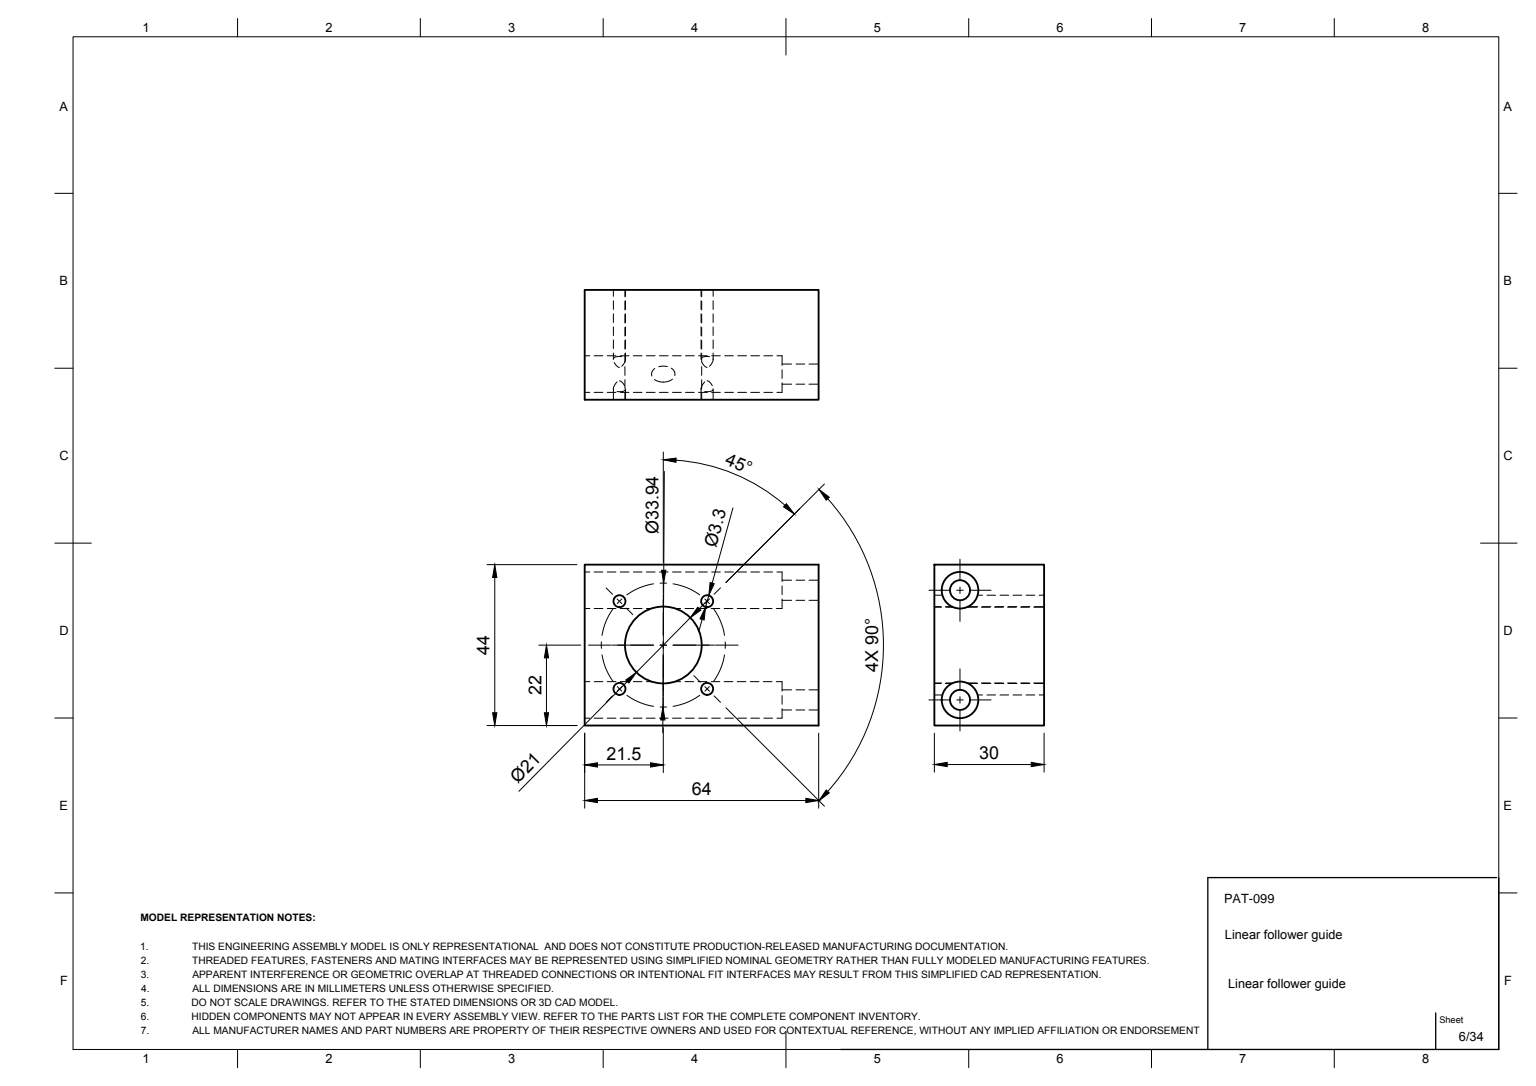
ISO-10303-21;
HEADER;
/* Generated by software containing ST-Developer
 * from STEP Tools, Inc. (www.steptools.com) 
 */

FILE_DESCRIPTION(
/* description */ ('PAT-099'),
/* implementation_level */ '2;1');

FILE_NAME(
/* name */ 'Linear follower guide.step',
/* time_stamp */ '2026-10-29T17:25:42-07:00',
/* author */ (''),
/* organization */ (''),
/* preprocessor_version */ 'ST-DEVELOPER v20.2',
/* originating_system */ 'Autodesk Translation Framework v15.17.0.0',
/* authorisation */ '');

FILE_SCHEMA (('AUTOMOTIVE_DESIGN { 1 0 10303 214 3 1 1 }'));
ENDSEC;

DATA;
#10=MECHANICAL_DESIGN_GEOMETRIC_PRESENTATION_REPRESENTATION('',(#338),#11035);
#241=B_SPLINE_CURVE_WITH_KNOTS('',3,(#7321,#7322,#7323,#7324,#7325,#7326,
#7327,#7328,#7329,#7330,#7331,#7332,#7333,#7334,#7335,#7336,#7337,#7338,
#7339,#7340,#7341,#7342,#7343,#7344,#7345,#7346,#7347,#7348,#7349,#7350),
 .UNSPECIFIED.,.F.,.F.,(4,2,2,2,2,2,2,2,2,2,2,2,2,2,4),(0.,0.0614386993115687,
0.122877398623137,0.194452004299172,0.266026609975207,0.361453659820112,
0.456880709665017,0.528368337752035,0.564112151795545,0.599855965839054,
0.635599779882563,0.671343593926072,0.742831222013091,0.838258271857996,
0.933685321702901),.UNSPECIFIED.);
#242=B_SPLINE_CURVE_WITH_KNOTS('',3,(#7351,#7352,#7353,#7354,#7355,#7356,
#7357,#7358,#7359,#7360),.UNSPECIFIED.,.F.,.F.,(4,2,2,2,4),(0.933685321702901,
1.00525992737894,1.07683453305497,1.13827323236654,1.19971193167811),
 .UNSPECIFIED.);
#243=B_SPLINE_CURVE_WITH_KNOTS('',3,(#7364,#7365,#7366,#7367,#7368,#7369,
#7370,#7371,#7372,#7373),.UNSPECIFIED.,.F.,.F.,(4,2,2,2,4),(0.,0.061438699311569,
0.122877398623138,0.194452004299173,0.266026609975207),.UNSPECIFIED.);
#244=B_SPLINE_CURVE_WITH_KNOTS('',3,(#7374,#7375,#7376,#7377,#7378,#7379,
#7380,#7381,#7382,#7383,#7384,#7385,#7386,#7387,#7388,#7389,#7390,#7391,
#7392,#7393,#7394,#7395,#7396,#7397,#7398,#7399,#7400,#7401,#7402,#7403),
 .UNSPECIFIED.,.F.,.F.,(4,2,2,2,2,2,2,2,2,2,2,2,2,2,4),(0.266026609975207,
0.361453659820112,0.456880709665017,0.528368337752036,0.564112151795545,
0.599855965839054,0.635599779882563,0.671343593926073,0.742831222013091,
0.838258271857996,0.933685321702901,1.00525992737894,1.07683453305497,1.13827323236654,
1.19971193167811),.UNSPECIFIED.);
#245=B_SPLINE_CURVE_WITH_KNOTS('',3,(#7413,#7414,#7415,#7416,#7417,#7418,
#7419,#7420,#7421,#7422,#7423,#7424,#7425,#7426,#7427,#7428,#7429,#7430,
#7431,#7432,#7433,#7434,#7435,#7436,#7437,#7438,#7439,#7440),
 .UNSPECIFIED.,.F.,.F.,(4,2,2,2,2,2,2,2,2,2,2,2,2,4),(0.,0.028138639371576,
0.0562772787431521,0.154843288866037,0.240109193198138,0.325375097530239,
0.395403587057064,0.46543207658389,0.528409281202622,0.591386485821355,
0.652825185132924,0.714263884444493,0.785838490120527,0.857413095796562),
 .UNSPECIFIED.);
#246=B_SPLINE_CURVE_WITH_KNOTS('',3,(#7441,#7442,#7443,#7444,#7445,#7446,
#7447,#7448,#7449,#7450,#7451,#7452),.UNSPECIFIED.,.F.,.F.,(4,2,2,2,2,4),
(0.857413095796562,0.952840145641466,1.04826719548637,1.11975482357339,
1.1554986376169,1.19124245166041),.UNSPECIFIED.);
#247=B_SPLINE_CURVE_WITH_KNOTS('',3,(#7456,#7457,#7458,#7459,#7460,#7461,
#7462,#7463,#7464,#7465,#7466,#7467),.UNSPECIFIED.,.F.,.F.,(4,2,2,2,2,4),
(0.,0.0357438140435093,0.0714876280870186,0.142975256174037,0.238402306018942,
0.333829355863846),.UNSPECIFIED.);
#248=B_SPLINE_CURVE_WITH_KNOTS('',3,(#7468,#7469,#7470,#7471,#7472,#7473,
#7474,#7475,#7476,#7477,#7478,#7479,#7480,#7481,#7482,#7483,#7484,#7485,
#7486,#7487,#7488,#7489,#7490,#7491,#7492,#7493,#7494,#7495),
 .UNSPECIFIED.,.F.,.F.,(4,2,2,2,2,2,2,2,2,2,2,2,2,4),(0.333829355863846,
0.40540396153988,0.476978567215915,0.538417266527484,0.599855965839053,
0.662833170457785,0.725810375076518,0.795838864603343,0.865867354130168,
0.951133258462269,1.03639916279437,1.13496517291726,1.16310381228883,1.19124245166041),
 .UNSPECIFIED.);
#249=B_SPLINE_CURVE_WITH_KNOTS('',3,(#7505,#7506,#7507,#7508,#7509,#7510,
#7511,#7512,#7513,#7514,#7515,#7516,#7517,#7518,#7519,#7520,#7521,#7522,
#7523,#7524,#7525,#7526,#7527,#7528,#7529,#7530,#7531,#7532),
 .UNSPECIFIED.,.F.,.F.,(4,2,2,2,2,2,2,2,2,2,2,2,2,4),(0.,0.0357438140435092,
0.0714876280870185,0.142975256174037,0.238402306018942,0.333829355863847,
0.405403961539882,0.476978567215916,0.538417266527485,0.599855965839054,
0.661294665150623,0.722733364462192,0.794307970138227,0.865882575814261),
 .UNSPECIFIED.);
#250=B_SPLINE_CURVE_WITH_KNOTS('',3,(#7533,#7534,#7535,#7536,#7537,#7538,
#7539,#7540,#7541,#7542,#7543,#7544),.UNSPECIFIED.,.F.,.F.,(4,2,2,2,2,4),
(0.865882575814261,0.961309625659166,1.05673667550407,1.12822430359109,
1.1639681176346,1.19971193167811),.UNSPECIFIED.);
#251=B_SPLINE_CURVE_WITH_KNOTS('',3,(#7548,#7549,#7550,#7551,#7552,#7553,
#7554,#7555,#7556,#7557,#7558,#7559),.UNSPECIFIED.,.F.,.F.,(4,2,2,2,2,4),
(0.,0.0357438140435093,0.0714876280870185,0.142975256174037,0.238402306018942,
0.333829355863847),.UNSPECIFIED.);
#252=B_SPLINE_CURVE_WITH_KNOTS('',3,(#7560,#7561,#7562,#7563,#7564,#7565,
#7566,#7567,#7568,#7569,#7570,#7571,#7572,#7573,#7574,#7575,#7576,#7577,
#7578,#7579,#7580,#7581,#7582,#7583,#7584,#7585,#7586,#7587),
 .UNSPECIFIED.,.F.,.F.,(4,2,2,2,2,2,2,2,2,2,2,2,2,4),(0.333829355863847,
0.405403961539881,0.476978567215916,0.538417266527485,0.599855965839054,
0.661294665150623,0.722733364462191,0.794307970138226,0.865882575814261,
0.961309625659166,1.05673667550407,1.12822430359109,1.1639681176346,1.19971193167811),
 .UNSPECIFIED.);
#253=B_SPLINE_CURVE_WITH_KNOTS('',3,(#7597,#7598,#7599,#7600,#7601,#7602,
#7603,#7604,#7605,#7606,#7607,#7608,#7609,#7610,#7611,#7612,#7613,#7614,
#7615,#7616,#7617,#7618,#7619,#7620,#7621,#7622,#7623,#7624,#7625,#7626),
 .UNSPECIFIED.,.F.,.F.,(4,2,2,2,2,2,2,2,2,2,2,2,2,2,4),(0.,0.0629772046187326,
0.125954409237465,0.195982898764291,0.266011388291116,0.351277292623217,
0.436543196955317,0.535109207078203,0.563247846449779,0.591386485821355,
0.627130299864864,0.662874113908373,0.734361741995392,0.829788791840296,
0.925215841685201),.UNSPECIFIED.);
#254=B_SPLINE_CURVE_WITH_KNOTS('',3,(#7627,#7628,#7629,#7630,#7631,#7632,
#7633,#7634,#7635,#7636),.UNSPECIFIED.,.F.,.F.,(4,2,2,2,4),(0.925215841685201,
0.996790447361235,1.06836505303727,1.12980375234884,1.19124245166041),
 .UNSPECIFIED.);
#255=B_SPLINE_CURVE_WITH_KNOTS('',3,(#7640,#7641,#7642,#7643,#7644,#7645,
#7646,#7647,#7648,#7649),.UNSPECIFIED.,.F.,.F.,(4,2,2,2,4),(0.,0.061438699311569,
0.122877398623138,0.194452004299172,0.266026609975207),.UNSPECIFIED.);
#256=B_SPLINE_CURVE_WITH_KNOTS('',3,(#7650,#7651,#7652,#7653,#7654,#7655,
#7656,#7657,#7658,#7659,#7660,#7661,#7662,#7663,#7664,#7665,#7666,#7667,
#7668,#7669,#7670,#7671,#7672,#7673,#7674,#7675,#7676,#7677,#7678,#7679),
 .UNSPECIFIED.,.F.,.F.,(4,2,2,2,2,2,2,2,2,2,2,2,2,2,4),(0.266026609975207,
0.361453659820111,0.456880709665016,0.528368337752034,0.564112151795544,
0.599855965839053,0.627994605210629,0.656133244582205,0.75469925470509,
0.839965159037191,0.925231063369292,0.995259552896117,1.06528804242294,
1.12826524704167,1.19124245166041),.UNSPECIFIED.);
#257=B_SPLINE_CURVE_WITH_KNOTS('',3,(#7688,#7689,#7690,#7691,#7692,#7693,
#7694,#7695,#7696,#7697,#7698,#7699,#7700,#7701,#7702,#7703,#7704,#7705,
#7706,#7707,#7708,#7709,#7710,#7711,#7712,#7713,#7714,#7715,#7716,#7717,
#7718,#7719,#7720,#7721,#7722,#7723,#7724,#7725,#7726,#7727,#7728,#7729),
 .UNSPECIFIED.,.T.,.F.,(4,2,2,2,2,2,2,2,2,2,2,2,2,2,2,2,2,2,2,2,4),(0.,
0.157447434703095,0.236171152054642,0.314894869406189,0.367076252690622,
0.419257635975055,0.471439019259488,0.523620402543921,0.602344119895468,
0.681067837247015,0.83851527195011,0.995962706653205,1.07468642400475,1.1534101413563,
1.20559152464073,1.25777290792516,1.3099542912096,1.36213567449403,1.44085939184558,
1.51958310919713,1.67703054390022),.UNSPECIFIED.);
#258=B_SPLINE_CURVE_WITH_KNOTS('',3,(#7742,#7743,#7744,#7745,#7746,#7747,
#7748,#7749,#7750,#7751,#7752,#7753,#7754,#7755,#7756,#7757,#7758,#7759,
#7760,#7761,#7762,#7763,#7764,#7765,#7766,#7767,#7768,#7769,#7770,#7771,
#7772,#7773,#7774,#7775,#7776,#7777,#7778,#7779,#7780,#7781,#7782,#7783),
 .UNSPECIFIED.,.T.,.F.,(4,2,2,2,2,2,2,2,2,2,2,2,2,2,2,2,2,2,2,2,4),(0.,
0.157447434703095,0.236171152054642,0.314894869406189,0.367076252690622,
0.419257635975055,0.471439019259488,0.523620402543921,0.602344119895468,
0.681067837247015,0.83851527195011,0.995962706653205,1.07468642400475,1.1534101413563,
1.20559152464073,1.25777290792516,1.3099542912096,1.36213567449403,1.44085939184558,
1.51958310919713,1.67703054390022),.UNSPECIFIED.);
#288=SHAPE_REPRESENTATION_RELATIONSHIP('SRR','None',#11156,#313);
#313=ADVANCED_BREP_SHAPE_REPRESENTATION('',(#371),#11006);
#338=STYLED_ITEM('',(#11400),#371);
#371=MANIFOLD_SOLID_BREP('Body1',#4706);
#413=FACE_BOUND('',#965,.T.);
#414=FACE_BOUND('',#966,.T.);
#415=FACE_BOUND('',#978,.T.);
#416=FACE_BOUND('',#979,.T.);
#417=FACE_BOUND('',#980,.T.);
#418=FACE_BOUND('',#981,.T.);
#419=FACE_BOUND('',#982,.T.);
#420=FACE_BOUND('',#984,.T.);
#421=FACE_BOUND('',#987,.T.);
#422=FACE_BOUND('',#988,.T.);
#423=FACE_BOUND('',#989,.T.);
#424=FACE_BOUND('',#990,.T.);
#425=FACE_BOUND('',#991,.T.);
#426=FACE_BOUND('',#993,.T.);
#427=FACE_BOUND('',#996,.T.);
#428=FACE_BOUND('',#997,.T.);
#429=FACE_BOUND('',#999,.T.);
#430=FACE_BOUND('',#1000,.T.);
#431=FACE_BOUND('',#1001,.T.);
#432=FACE_BOUND('',#1002,.T.);
#433=FACE_BOUND('',#1003,.T.);
#434=FACE_BOUND('',#1005,.T.);
#435=FACE_BOUND('',#1006,.T.);
#436=FACE_BOUND('',#1007,.T.);
#437=FACE_BOUND('',#1008,.T.);
#438=FACE_BOUND('',#1009,.T.);
#439=FACE_BOUND('',#1011,.T.);
#440=FACE_BOUND('',#1012,.T.);
#529=PLANE('',#5044);
#530=PLANE('',#5047);
#531=PLANE('',#5048);
#532=PLANE('',#5067);
#533=PLANE('',#5073);
#534=PLANE('',#5080);
#535=PLANE('',#5081);
#536=PLANE('',#5082);
#671=FACE_OUTER_BOUND('',#964,.T.);
#672=FACE_OUTER_BOUND('',#967,.T.);
#673=FACE_OUTER_BOUND('',#968,.T.);
#674=FACE_OUTER_BOUND('',#969,.T.);
#675=FACE_OUTER_BOUND('',#970,.T.);
#676=FACE_OUTER_BOUND('',#971,.T.);
#677=FACE_OUTER_BOUND('',#972,.T.);
#678=FACE_OUTER_BOUND('',#973,.T.);
#679=FACE_OUTER_BOUND('',#974,.T.);
#680=FACE_OUTER_BOUND('',#975,.T.);
#681=FACE_OUTER_BOUND('',#976,.T.);
#682=FACE_OUTER_BOUND('',#977,.T.);
#683=FACE_OUTER_BOUND('',#983,.T.);
#684=FACE_OUTER_BOUND('',#985,.T.);
#685=FACE_OUTER_BOUND('',#986,.T.);
#686=FACE_OUTER_BOUND('',#992,.T.);
#687=FACE_OUTER_BOUND('',#994,.T.);
#688=FACE_OUTER_BOUND('',#995,.T.);
#689=FACE_OUTER_BOUND('',#998,.T.);
#690=FACE_OUTER_BOUND('',#1004,.T.);
#691=FACE_OUTER_BOUND('',#1010,.T.);
#964=EDGE_LOOP('',(#3191,#3192,#3193,#3194));
#965=EDGE_LOOP('',(#3195));
#966=EDGE_LOOP('',(#3196));
#967=EDGE_LOOP('',(#3197,#3198,#3199,#3200));
#968=EDGE_LOOP('',(#3201,#3202,#3203,#3204));
#969=EDGE_LOOP('',(#3205,#3206,#3207,#3208,#3209));
#970=EDGE_LOOP('',(#3210,#3211,#3212,#3213,#3214));
#971=EDGE_LOOP('',(#3215,#3216,#3217,#3218,#3219));
#972=EDGE_LOOP('',(#3220,#3221,#3222,#3223,#3224));
#973=EDGE_LOOP('',(#3225,#3226,#3227,#3228,#3229));
#974=EDGE_LOOP('',(#3230,#3231,#3232,#3233,#3234));
#975=EDGE_LOOP('',(#3235,#3236,#3237,#3238,#3239));
#976=EDGE_LOOP('',(#3240,#3241,#3242,#3243,#3244));
#977=EDGE_LOOP('',(#3245,#3246,#3247,#3248));
#978=EDGE_LOOP('',(#3249,#3250));
#979=EDGE_LOOP('',(#3251,#3252));
#980=EDGE_LOOP('',(#3253,#3254));
#981=EDGE_LOOP('',(#3255,#3256));
#982=EDGE_LOOP('',(#3257));
#983=EDGE_LOOP('',(#3258));
#984=EDGE_LOOP('',(#3259));
#985=EDGE_LOOP('',(#3260,#3261,#3262,#3263));
#986=EDGE_LOOP('',(#3264,#3265,#3266,#3267));
#987=EDGE_LOOP('',(#3268,#3269));
#988=EDGE_LOOP('',(#3270,#3271));
#989=EDGE_LOOP('',(#3272,#3273));
#990=EDGE_LOOP('',(#3274,#3275));
#991=EDGE_LOOP('',(#3276));
#992=EDGE_LOOP('',(#3277));
#993=EDGE_LOOP('',(#3278));
#994=EDGE_LOOP('',(#3279,#3280,#3281,#3282));
#995=EDGE_LOOP('',(#3283,#3284,#3285,#3286));
#996=EDGE_LOOP('',(#3287));
#997=EDGE_LOOP('',(#3288));
#998=EDGE_LOOP('',(#3289,#3290,#3291,#3292));
#999=EDGE_LOOP('',(#3293));
#1000=EDGE_LOOP('',(#3294));
#1001=EDGE_LOOP('',(#3295));
#1002=EDGE_LOOP('',(#3296));
#1003=EDGE_LOOP('',(#3297));
#1004=EDGE_LOOP('',(#3298,#3299,#3300,#3301));
#1005=EDGE_LOOP('',(#3302));
#1006=EDGE_LOOP('',(#3303));
#1007=EDGE_LOOP('',(#3304));
#1008=EDGE_LOOP('',(#3305));
#1009=EDGE_LOOP('',(#3306));
#1010=EDGE_LOOP('',(#3307,#3308,#3309,#3310));
#1011=EDGE_LOOP('',(#3311));
#1012=EDGE_LOOP('',(#3312));
#1361=LINE('',#7293,#1613);
#1362=LINE('',#7295,#1614);
#1363=LINE('',#7297,#1615);
#1364=LINE('',#7298,#1616);
#1365=LINE('',#7306,#1617);
#1366=LINE('',#7307,#1618);
#1367=LINE('',#7308,#1619);
#1368=LINE('',#7312,#1620);
#1369=LINE('',#7313,#1621);
#1370=LINE('',#7314,#1622);
#1371=LINE('',#7319,#1623);
#1372=LINE('',#7405,#1624);
#1373=LINE('',#7411,#1625);
#1374=LINE('',#7497,#1626);
#1375=LINE('',#7503,#1627);
#1376=LINE('',#7589,#1628);
#1377=LINE('',#7595,#1629);
#1378=LINE('',#7681,#1630);
#1379=LINE('',#7686,#1631);
#1380=LINE('',#7736,#1632);
#1381=LINE('',#7740,#1633);
#1382=LINE('',#7790,#1634);
#1383=LINE('',#7795,#1635);
#1384=LINE('',#7798,#1636);
#1385=LINE('',#7800,#1637);
#1613=VECTOR('',#5744,1.);
#1614=VECTOR('',#5745,1.);
#1615=VECTOR('',#5746,1.);
#1616=VECTOR('',#5747,1.);
#1617=VECTOR('',#5754,1.);
#1618=VECTOR('',#5755,1.);
#1619=VECTOR('',#5756,1.);
#1620=VECTOR('',#5759,1.);
#1621=VECTOR('',#5760,1.);
#1622=VECTOR('',#5761,1.);
#1623=VECTOR('',#5766,0.165);
#1624=VECTOR('',#5769,0.165);
#1625=VECTOR('',#5776,0.165);
#1626=VECTOR('',#5779,0.165);
#1627=VECTOR('',#5786,0.165);
#1628=VECTOR('',#5789,0.165);
#1629=VECTOR('',#5796,0.165);
#1630=VECTOR('',#5799,0.165);
#1631=VECTOR('',#5806,0.5);
#1632=VECTOR('',#5815,0.275);
#1633=VECTOR('',#5820,0.5);
#1634=VECTOR('',#5829,0.275);
#1635=VECTOR('',#5834,1.05);
#1636=VECTOR('',#5839,1.);
#1637=VECTOR('',#5842,1.);
#1859=CIRCLE('',#5045,0.5);
#1860=CIRCLE('',#5046,0.5);
#1861=CIRCLE('',#5050,0.165);
#1862=CIRCLE('',#5052,0.165);
#1863=CIRCLE('',#5054,0.165);
#1864=CIRCLE('',#5056,0.165);
#1865=CIRCLE('',#5058,0.165);
#1866=CIRCLE('',#5060,0.165);
#1867=CIRCLE('',#5062,0.165);
#1868=CIRCLE('',#5064,0.165);
#1869=CIRCLE('',#5066,0.5);
#1870=CIRCLE('',#5068,0.275);
#1871=CIRCLE('',#5070,0.275);
#1872=CIRCLE('',#5072,0.5);
#1873=CIRCLE('',#5074,0.275);
#1874=CIRCLE('',#5076,0.275);
#1875=CIRCLE('',#5078,1.05);
#1876=CIRCLE('',#5079,1.05);
#2158=VERTEX_POINT('',#7291);
#2159=VERTEX_POINT('',#7292);
#2160=VERTEX_POINT('',#7294);
#2161=VERTEX_POINT('',#7296);
#2162=VERTEX_POINT('',#7299);
#2163=VERTEX_POINT('',#7301);
#2164=VERTEX_POINT('',#7304);
#2165=VERTEX_POINT('',#7305);
#2166=VERTEX_POINT('',#7310);
#2167=VERTEX_POINT('',#7311);
#2168=VERTEX_POINT('',#7316);
#2169=VERTEX_POINT('',#7318);
#2170=VERTEX_POINT('',#7320);
#2171=VERTEX_POINT('',#7362);
#2172=VERTEX_POINT('',#7363);
#2173=VERTEX_POINT('',#7404);
#2174=VERTEX_POINT('',#7408);
#2175=VERTEX_POINT('',#7410);
#2176=VERTEX_POINT('',#7412);
#2177=VERTEX_POINT('',#7454);
#2178=VERTEX_POINT('',#7455);
#2179=VERTEX_POINT('',#7496);
#2180=VERTEX_POINT('',#7500);
#2181=VERTEX_POINT('',#7502);
#2182=VERTEX_POINT('',#7504);
#2183=VERTEX_POINT('',#7546);
#2184=VERTEX_POINT('',#7547);
#2185=VERTEX_POINT('',#7588);
#2186=VERTEX_POINT('',#7592);
#2187=VERTEX_POINT('',#7594);
#2188=VERTEX_POINT('',#7596);
#2189=VERTEX_POINT('',#7638);
#2190=VERTEX_POINT('',#7639);
#2191=VERTEX_POINT('',#7680);
#2192=VERTEX_POINT('',#7684);
#2193=VERTEX_POINT('',#7687);
#2194=VERTEX_POINT('',#7731);
#2195=VERTEX_POINT('',#7734);
#2196=VERTEX_POINT('',#7738);
#2197=VERTEX_POINT('',#7741);
#2198=VERTEX_POINT('',#7785);
#2199=VERTEX_POINT('',#7788);
#2200=VERTEX_POINT('',#7792);
#2201=VERTEX_POINT('',#7794);
#2572=EDGE_CURVE('',#2158,#2159,#1361,.T.);
#2573=EDGE_CURVE('',#2159,#2160,#1362,.T.);
#2574=EDGE_CURVE('',#2160,#2161,#1363,.T.);
#2575=EDGE_CURVE('',#2161,#2158,#1364,.T.);
#2576=EDGE_CURVE('',#2162,#2162,#1859,.T.);
#2577=EDGE_CURVE('',#2163,#2163,#1860,.T.);
#2578=EDGE_CURVE('',#2164,#2165,#1365,.T.);
#2579=EDGE_CURVE('',#2165,#2158,#1366,.T.);
#2580=EDGE_CURVE('',#2164,#2161,#1367,.T.);
#2581=EDGE_CURVE('',#2166,#2167,#1368,.T.);
#2582=EDGE_CURVE('',#2167,#2160,#1369,.T.);
#2583=EDGE_CURVE('',#2166,#2159,#1370,.T.);
#2584=EDGE_CURVE('',#2168,#2168,#1861,.T.);
#2585=EDGE_CURVE('',#2168,#2169,#1371,.T.);
#2586=EDGE_CURVE('',#2170,#2169,#241,.T.);
#2587=EDGE_CURVE('',#2169,#2170,#242,.T.);
#2588=EDGE_CURVE('',#2171,#2172,#243,.T.);
#2589=EDGE_CURVE('',#2172,#2171,#244,.T.);
#2590=EDGE_CURVE('',#2172,#2173,#1372,.T.);
#2591=EDGE_CURVE('',#2173,#2173,#1862,.T.);
#2592=EDGE_CURVE('',#2174,#2174,#1863,.T.);
#2593=EDGE_CURVE('',#2174,#2175,#1373,.T.);
#2594=EDGE_CURVE('',#2176,#2175,#245,.T.);
#2595=EDGE_CURVE('',#2175,#2176,#246,.T.);
#2596=EDGE_CURVE('',#2177,#2178,#247,.T.);
#2597=EDGE_CURVE('',#2178,#2177,#248,.T.);
#2598=EDGE_CURVE('',#2178,#2179,#1374,.T.);
#2599=EDGE_CURVE('',#2179,#2179,#1864,.T.);
#2600=EDGE_CURVE('',#2180,#2180,#1865,.T.);
#2601=EDGE_CURVE('',#2180,#2181,#1375,.T.);
#2602=EDGE_CURVE('',#2182,#2181,#249,.T.);
#2603=EDGE_CURVE('',#2181,#2182,#250,.T.);
#2604=EDGE_CURVE('',#2183,#2184,#251,.T.);
#2605=EDGE_CURVE('',#2184,#2183,#252,.T.);
#2606=EDGE_CURVE('',#2184,#2185,#1376,.T.);
#2607=EDGE_CURVE('',#2185,#2185,#1866,.T.);
#2608=EDGE_CURVE('',#2186,#2186,#1867,.T.);
#2609=EDGE_CURVE('',#2186,#2187,#1377,.T.);
#2610=EDGE_CURVE('',#2188,#2187,#253,.T.);
#2611=EDGE_CURVE('',#2187,#2188,#254,.T.);
#2612=EDGE_CURVE('',#2189,#2190,#255,.T.);
#2613=EDGE_CURVE('',#2190,#2189,#256,.T.);
#2614=EDGE_CURVE('',#2190,#2191,#1378,.T.);
#2615=EDGE_CURVE('',#2191,#2191,#1868,.T.);
#2616=EDGE_CURVE('',#2192,#2192,#1869,.T.);
#2617=EDGE_CURVE('',#2192,#2162,#1379,.T.);
#2618=EDGE_CURVE('',#2193,#2193,#257,.T.);
#2619=EDGE_CURVE('',#2194,#2194,#1870,.T.);
#2620=EDGE_CURVE('',#2195,#2195,#1871,.T.);
#2621=EDGE_CURVE('',#2195,#2194,#1380,.T.);
#2622=EDGE_CURVE('',#2196,#2196,#1872,.T.);
#2623=EDGE_CURVE('',#2196,#2163,#1381,.T.);
#2624=EDGE_CURVE('',#2197,#2197,#258,.T.);
#2625=EDGE_CURVE('',#2198,#2198,#1873,.T.);
#2626=EDGE_CURVE('',#2199,#2199,#1874,.T.);
#2627=EDGE_CURVE('',#2199,#2198,#1382,.T.);
#2628=EDGE_CURVE('',#2200,#2200,#1875,.T.);
#2629=EDGE_CURVE('',#2200,#2201,#1383,.T.);
#2630=EDGE_CURVE('',#2201,#2201,#1876,.T.);
#2631=EDGE_CURVE('',#2164,#2167,#1384,.T.);
#2632=EDGE_CURVE('',#2165,#2166,#1385,.T.);
#3191=ORIENTED_EDGE('',*,*,#2572,.T.);
#3192=ORIENTED_EDGE('',*,*,#2573,.T.);
#3193=ORIENTED_EDGE('',*,*,#2574,.T.);
#3194=ORIENTED_EDGE('',*,*,#2575,.T.);
#3195=ORIENTED_EDGE('',*,*,#2576,.T.);
#3196=ORIENTED_EDGE('',*,*,#2577,.T.);
#3197=ORIENTED_EDGE('',*,*,#2578,.T.);
#3198=ORIENTED_EDGE('',*,*,#2579,.T.);
#3199=ORIENTED_EDGE('',*,*,#2575,.F.);
#3200=ORIENTED_EDGE('',*,*,#2580,.F.);
#3201=ORIENTED_EDGE('',*,*,#2581,.T.);
#3202=ORIENTED_EDGE('',*,*,#2582,.T.);
#3203=ORIENTED_EDGE('',*,*,#2573,.F.);
#3204=ORIENTED_EDGE('',*,*,#2583,.F.);
#3205=ORIENTED_EDGE('',*,*,#2584,.F.);
#3206=ORIENTED_EDGE('',*,*,#2585,.T.);
#3207=ORIENTED_EDGE('',*,*,#2586,.F.);
#3208=ORIENTED_EDGE('',*,*,#2587,.F.);
#3209=ORIENTED_EDGE('',*,*,#2585,.F.);
#3210=ORIENTED_EDGE('',*,*,#2588,.F.);
#3211=ORIENTED_EDGE('',*,*,#2589,.F.);
#3212=ORIENTED_EDGE('',*,*,#2590,.T.);
#3213=ORIENTED_EDGE('',*,*,#2591,.F.);
#3214=ORIENTED_EDGE('',*,*,#2590,.F.);
#3215=ORIENTED_EDGE('',*,*,#2592,.F.);
#3216=ORIENTED_EDGE('',*,*,#2593,.T.);
#3217=ORIENTED_EDGE('',*,*,#2594,.F.);
#3218=ORIENTED_EDGE('',*,*,#2595,.F.);
#3219=ORIENTED_EDGE('',*,*,#2593,.F.);
#3220=ORIENTED_EDGE('',*,*,#2596,.F.);
#3221=ORIENTED_EDGE('',*,*,#2597,.F.);
#3222=ORIENTED_EDGE('',*,*,#2598,.T.);
#3223=ORIENTED_EDGE('',*,*,#2599,.F.);
#3224=ORIENTED_EDGE('',*,*,#2598,.F.);
#3225=ORIENTED_EDGE('',*,*,#2600,.F.);
#3226=ORIENTED_EDGE('',*,*,#2601,.T.);
#3227=ORIENTED_EDGE('',*,*,#2602,.F.);
#3228=ORIENTED_EDGE('',*,*,#2603,.F.);
#3229=ORIENTED_EDGE('',*,*,#2601,.F.);
#3230=ORIENTED_EDGE('',*,*,#2604,.F.);
#3231=ORIENTED_EDGE('',*,*,#2605,.F.);
#3232=ORIENTED_EDGE('',*,*,#2606,.T.);
#3233=ORIENTED_EDGE('',*,*,#2607,.F.);
#3234=ORIENTED_EDGE('',*,*,#2606,.F.);
#3235=ORIENTED_EDGE('',*,*,#2608,.F.);
#3236=ORIENTED_EDGE('',*,*,#2609,.T.);
#3237=ORIENTED_EDGE('',*,*,#2610,.F.);
#3238=ORIENTED_EDGE('',*,*,#2611,.F.);
#3239=ORIENTED_EDGE('',*,*,#2609,.F.);
#3240=ORIENTED_EDGE('',*,*,#2612,.F.);
#3241=ORIENTED_EDGE('',*,*,#2613,.F.);
#3242=ORIENTED_EDGE('',*,*,#2614,.T.);
#3243=ORIENTED_EDGE('',*,*,#2615,.F.);
#3244=ORIENTED_EDGE('',*,*,#2614,.F.);
#3245=ORIENTED_EDGE('',*,*,#2616,.F.);
#3246=ORIENTED_EDGE('',*,*,#2617,.T.);
#3247=ORIENTED_EDGE('',*,*,#2576,.F.);
#3248=ORIENTED_EDGE('',*,*,#2617,.F.);
#3249=ORIENTED_EDGE('',*,*,#2588,.T.);
#3250=ORIENTED_EDGE('',*,*,#2589,.T.);
#3251=ORIENTED_EDGE('',*,*,#2586,.T.);
#3252=ORIENTED_EDGE('',*,*,#2587,.T.);
#3253=ORIENTED_EDGE('',*,*,#2612,.T.);
#3254=ORIENTED_EDGE('',*,*,#2613,.T.);
#3255=ORIENTED_EDGE('',*,*,#2610,.T.);
#3256=ORIENTED_EDGE('',*,*,#2611,.T.);
#3257=ORIENTED_EDGE('',*,*,#2618,.F.);
#3258=ORIENTED_EDGE('',*,*,#2616,.T.);
#3259=ORIENTED_EDGE('',*,*,#2619,.F.);
#3260=ORIENTED_EDGE('',*,*,#2620,.F.);
#3261=ORIENTED_EDGE('',*,*,#2621,.T.);
#3262=ORIENTED_EDGE('',*,*,#2619,.T.);
#3263=ORIENTED_EDGE('',*,*,#2621,.F.);
#3264=ORIENTED_EDGE('',*,*,#2622,.F.);
#3265=ORIENTED_EDGE('',*,*,#2623,.T.);
#3266=ORIENTED_EDGE('',*,*,#2577,.F.);
#3267=ORIENTED_EDGE('',*,*,#2623,.F.);
#3268=ORIENTED_EDGE('',*,*,#2596,.T.);
#3269=ORIENTED_EDGE('',*,*,#2597,.T.);
#3270=ORIENTED_EDGE('',*,*,#2594,.T.);
#3271=ORIENTED_EDGE('',*,*,#2595,.T.);
#3272=ORIENTED_EDGE('',*,*,#2604,.T.);
#3273=ORIENTED_EDGE('',*,*,#2605,.T.);
#3274=ORIENTED_EDGE('',*,*,#2602,.T.);
#3275=ORIENTED_EDGE('',*,*,#2603,.T.);
#3276=ORIENTED_EDGE('',*,*,#2624,.F.);
#3277=ORIENTED_EDGE('',*,*,#2622,.T.);
#3278=ORIENTED_EDGE('',*,*,#2625,.F.);
#3279=ORIENTED_EDGE('',*,*,#2626,.F.);
#3280=ORIENTED_EDGE('',*,*,#2627,.T.);
#3281=ORIENTED_EDGE('',*,*,#2625,.T.);
#3282=ORIENTED_EDGE('',*,*,#2627,.F.);
#3283=ORIENTED_EDGE('',*,*,#2628,.F.);
#3284=ORIENTED_EDGE('',*,*,#2629,.T.);
#3285=ORIENTED_EDGE('',*,*,#2630,.F.);
#3286=ORIENTED_EDGE('',*,*,#2629,.F.);
#3287=ORIENTED_EDGE('',*,*,#2618,.T.);
#3288=ORIENTED_EDGE('',*,*,#2624,.T.);
#3289=ORIENTED_EDGE('',*,*,#2631,.F.);
#3290=ORIENTED_EDGE('',*,*,#2580,.T.);
#3291=ORIENTED_EDGE('',*,*,#2574,.F.);
#3292=ORIENTED_EDGE('',*,*,#2582,.F.);
#3293=ORIENTED_EDGE('',*,*,#2630,.T.);
#3294=ORIENTED_EDGE('',*,*,#2615,.T.);
#3295=ORIENTED_EDGE('',*,*,#2607,.T.);
#3296=ORIENTED_EDGE('',*,*,#2599,.T.);
#3297=ORIENTED_EDGE('',*,*,#2591,.T.);
#3298=ORIENTED_EDGE('',*,*,#2632,.T.);
#3299=ORIENTED_EDGE('',*,*,#2583,.T.);
#3300=ORIENTED_EDGE('',*,*,#2572,.F.);
#3301=ORIENTED_EDGE('',*,*,#2579,.F.);
#3302=ORIENTED_EDGE('',*,*,#2628,.T.);
#3303=ORIENTED_EDGE('',*,*,#2608,.T.);
#3304=ORIENTED_EDGE('',*,*,#2600,.T.);
#3305=ORIENTED_EDGE('',*,*,#2592,.T.);
#3306=ORIENTED_EDGE('',*,*,#2584,.T.);
#3307=ORIENTED_EDGE('',*,*,#2632,.F.);
#3308=ORIENTED_EDGE('',*,*,#2578,.F.);
#3309=ORIENTED_EDGE('',*,*,#2631,.T.);
#3310=ORIENTED_EDGE('',*,*,#2581,.F.);
#3311=ORIENTED_EDGE('',*,*,#2620,.T.);
#3312=ORIENTED_EDGE('',*,*,#2626,.T.);
#4315=CYLINDRICAL_SURFACE('',#5049,0.165);
#4316=CYLINDRICAL_SURFACE('',#5051,0.165);
#4317=CYLINDRICAL_SURFACE('',#5053,0.165);
#4318=CYLINDRICAL_SURFACE('',#5055,0.165);
#4319=CYLINDRICAL_SURFACE('',#5057,0.165);
#4320=CYLINDRICAL_SURFACE('',#5059,0.165);
#4321=CYLINDRICAL_SURFACE('',#5061,0.165);
#4322=CYLINDRICAL_SURFACE('',#5063,0.165);
#4323=CYLINDRICAL_SURFACE('',#5065,0.5);
#4324=CYLINDRICAL_SURFACE('',#5069,0.275);
#4325=CYLINDRICAL_SURFACE('',#5071,0.5);
#4326=CYLINDRICAL_SURFACE('',#5075,0.275);
#4327=CYLINDRICAL_SURFACE('',#5077,1.05);
#4436=ADVANCED_FACE('',(#671,#413,#414),#529,.T.);
#4437=ADVANCED_FACE('',(#672),#530,.T.);
#4438=ADVANCED_FACE('',(#673),#531,.T.);
#4439=ADVANCED_FACE('',(#674),#4315,.F.);
#4440=ADVANCED_FACE('',(#675),#4316,.F.);
#4441=ADVANCED_FACE('',(#676),#4317,.F.);
#4442=ADVANCED_FACE('',(#677),#4318,.F.);
#4443=ADVANCED_FACE('',(#678),#4319,.F.);
#4444=ADVANCED_FACE('',(#679),#4320,.F.);
#4445=ADVANCED_FACE('',(#680),#4321,.F.);
#4446=ADVANCED_FACE('',(#681),#4322,.F.);
#4447=ADVANCED_FACE('',(#682,#415,#416,#417,#418,#419),#4323,.F.);
#4448=ADVANCED_FACE('',(#683,#420),#532,.T.);
#4449=ADVANCED_FACE('',(#684),#4324,.F.);
#4450=ADVANCED_FACE('',(#685,#421,#422,#423,#424,#425),#4325,.F.);
#4451=ADVANCED_FACE('',(#686,#426),#533,.T.);
#4452=ADVANCED_FACE('',(#687),#4326,.F.);
#4453=ADVANCED_FACE('',(#688,#427,#428),#4327,.F.);
#4454=ADVANCED_FACE('',(#689,#429,#430,#431,#432,#433),#534,.T.);
#4455=ADVANCED_FACE('',(#690,#434,#435,#436,#437,#438),#535,.T.);
#4456=ADVANCED_FACE('',(#691,#439,#440),#536,.F.);
#4706=CLOSED_SHELL('',(#4436,#4437,#4438,#4439,#4440,#4441,#4442,#4443,
#4444,#4445,#4446,#4447,#4448,#4449,#4450,#4451,#4452,#4453,#4454,#4455,
#4456));
#5043=AXIS2_PLACEMENT_3D('',#7289,#5740,#5741);
#5044=AXIS2_PLACEMENT_3D('',#7290,#5742,#5743);
#5045=AXIS2_PLACEMENT_3D('',#7300,#5748,#5749);
#5046=AXIS2_PLACEMENT_3D('',#7302,#5750,#5751);
#5047=AXIS2_PLACEMENT_3D('',#7303,#5752,#5753);
#5048=AXIS2_PLACEMENT_3D('',#7309,#5757,#5758);
#5049=AXIS2_PLACEMENT_3D('',#7315,#5762,#5763);
#5050=AXIS2_PLACEMENT_3D('',#7317,#5764,#5765);
#5051=AXIS2_PLACEMENT_3D('',#7361,#5767,#5768);
#5052=AXIS2_PLACEMENT_3D('',#7406,#5770,#5771);
#5053=AXIS2_PLACEMENT_3D('',#7407,#5772,#5773);
#5054=AXIS2_PLACEMENT_3D('',#7409,#5774,#5775);
#5055=AXIS2_PLACEMENT_3D('',#7453,#5777,#5778);
#5056=AXIS2_PLACEMENT_3D('',#7498,#5780,#5781);
#5057=AXIS2_PLACEMENT_3D('',#7499,#5782,#5783);
#5058=AXIS2_PLACEMENT_3D('',#7501,#5784,#5785);
#5059=AXIS2_PLACEMENT_3D('',#7545,#5787,#5788);
#5060=AXIS2_PLACEMENT_3D('',#7590,#5790,#5791);
#5061=AXIS2_PLACEMENT_3D('',#7591,#5792,#5793);
#5062=AXIS2_PLACEMENT_3D('',#7593,#5794,#5795);
#5063=AXIS2_PLACEMENT_3D('',#7637,#5797,#5798);
#5064=AXIS2_PLACEMENT_3D('',#7682,#5800,#5801);
#5065=AXIS2_PLACEMENT_3D('',#7683,#5802,#5803);
#5066=AXIS2_PLACEMENT_3D('',#7685,#5804,#5805);
#5067=AXIS2_PLACEMENT_3D('',#7730,#5807,#5808);
#5068=AXIS2_PLACEMENT_3D('',#7732,#5809,#5810);
#5069=AXIS2_PLACEMENT_3D('',#7733,#5811,#5812);
#5070=AXIS2_PLACEMENT_3D('',#7735,#5813,#5814);
#5071=AXIS2_PLACEMENT_3D('',#7737,#5816,#5817);
#5072=AXIS2_PLACEMENT_3D('',#7739,#5818,#5819);
#5073=AXIS2_PLACEMENT_3D('',#7784,#5821,#5822);
#5074=AXIS2_PLACEMENT_3D('',#7786,#5823,#5824);
#5075=AXIS2_PLACEMENT_3D('',#7787,#5825,#5826);
#5076=AXIS2_PLACEMENT_3D('',#7789,#5827,#5828);
#5077=AXIS2_PLACEMENT_3D('',#7791,#5830,#5831);
#5078=AXIS2_PLACEMENT_3D('',#7793,#5832,#5833);
#5079=AXIS2_PLACEMENT_3D('',#7796,#5835,#5836);
#5080=AXIS2_PLACEMENT_3D('',#7797,#5837,#5838);
#5081=AXIS2_PLACEMENT_3D('',#7799,#5840,#5841);
#5082=AXIS2_PLACEMENT_3D('',#7801,#5843,#5844);
#5740=DIRECTION('axis',(0.,0.,1.));
#5741=DIRECTION('refdir',(1.,0.,0.));
#5742=DIRECTION('center_axis',(0.,0.,1.));
#5743=DIRECTION('ref_axis',(1.,0.,0.));
#5744=DIRECTION('',(0.,-1.,0.));
#5745=DIRECTION('',(1.,0.,0.));
#5746=DIRECTION('',(0.,1.,0.));
#5747=DIRECTION('',(-1.,0.,0.));
#5748=DIRECTION('center_axis',(0.,0.,-1.));
#5749=DIRECTION('ref_axis',(1.,0.,0.));
#5750=DIRECTION('center_axis',(0.,0.,-1.));
#5751=DIRECTION('ref_axis',(1.,0.,0.));
#5752=DIRECTION('center_axis',(0.,1.,0.));
#5753=DIRECTION('ref_axis',(0.,0.,1.));
#5754=DIRECTION('',(-1.,0.,0.));
#5755=DIRECTION('',(0.,0.,1.));
#5756=DIRECTION('',(0.,0.,1.));
#5757=DIRECTION('center_axis',(0.,-1.,0.));
#5758=DIRECTION('ref_axis',(0.,0.,-1.));
#5759=DIRECTION('',(1.,0.,0.));
#5760=DIRECTION('',(0.,0.,1.));
#5761=DIRECTION('',(0.,0.,1.));
#5762=DIRECTION('center_axis',(1.,0.,0.));
#5763=DIRECTION('ref_axis',(0.,0.,-1.));
#5764=DIRECTION('center_axis',(1.,0.,0.));
#5765=DIRECTION('ref_axis',(0.,0.,-1.));
#5766=DIRECTION('',(1.,0.,0.));
#5767=DIRECTION('center_axis',(1.,0.,0.));
#5768=DIRECTION('ref_axis',(0.,0.,-1.));
#5769=DIRECTION('',(1.,0.,0.));
#5770=DIRECTION('center_axis',(-1.,0.,0.));
#5771=DIRECTION('ref_axis',(0.,0.,-1.));
#5772=DIRECTION('center_axis',(1.,0.,0.));
#5773=DIRECTION('ref_axis',(0.,0.,-1.));
#5774=DIRECTION('center_axis',(1.,0.,0.));
#5775=DIRECTION('ref_axis',(0.,0.,-1.));
#5776=DIRECTION('',(1.,0.,0.));
#5777=DIRECTION('center_axis',(1.,0.,0.));
#5778=DIRECTION('ref_axis',(0.,0.,-1.));
#5779=DIRECTION('',(1.,0.,0.));
#5780=DIRECTION('center_axis',(-1.,0.,0.));
#5781=DIRECTION('ref_axis',(0.,0.,-1.));
#5782=DIRECTION('center_axis',(1.,0.,0.));
#5783=DIRECTION('ref_axis',(0.,0.,-1.));
#5784=DIRECTION('center_axis',(1.,0.,0.));
#5785=DIRECTION('ref_axis',(0.,0.,-1.));
#5786=DIRECTION('',(1.,0.,0.));
#5787=DIRECTION('center_axis',(1.,0.,0.));
#5788=DIRECTION('ref_axis',(0.,0.,-1.));
#5789=DIRECTION('',(1.,0.,0.));
#5790=DIRECTION('center_axis',(-1.,0.,0.));
#5791=DIRECTION('ref_axis',(0.,0.,-1.));
#5792=DIRECTION('center_axis',(1.,0.,0.));
#5793=DIRECTION('ref_axis',(0.,0.,-1.));
#5794=DIRECTION('center_axis',(1.,0.,0.));
#5795=DIRECTION('ref_axis',(0.,0.,-1.));
#5796=DIRECTION('',(1.,0.,0.));
#5797=DIRECTION('center_axis',(1.,0.,0.));
#5798=DIRECTION('ref_axis',(0.,0.,-1.));
#5799=DIRECTION('',(1.,0.,0.));
#5800=DIRECTION('center_axis',(-1.,0.,0.));
#5801=DIRECTION('ref_axis',(0.,0.,-1.));
#5802=DIRECTION('center_axis',(0.,0.,1.));
#5803=DIRECTION('ref_axis',(1.,0.,0.));
#5804=DIRECTION('center_axis',(0.,0.,1.));
#5805=DIRECTION('ref_axis',(1.,0.,0.));
#5806=DIRECTION('',(0.,0.,1.));
#5807=DIRECTION('center_axis',(0.,0.,1.));
#5808=DIRECTION('ref_axis',(1.,0.,0.));
#5809=DIRECTION('center_axis',(0.,0.,1.));
#5810=DIRECTION('ref_axis',(1.,0.,0.));
#5811=DIRECTION('center_axis',(0.,0.,1.));
#5812=DIRECTION('ref_axis',(1.,0.,0.));
#5813=DIRECTION('center_axis',(0.,0.,1.));
#5814=DIRECTION('ref_axis',(1.,0.,0.));
#5815=DIRECTION('',(0.,0.,1.));
#5816=DIRECTION('center_axis',(0.,0.,1.));
#5817=DIRECTION('ref_axis',(1.,0.,0.));
#5818=DIRECTION('center_axis',(0.,0.,1.));
#5819=DIRECTION('ref_axis',(1.,0.,0.));
#5820=DIRECTION('',(0.,0.,1.));
#5821=DIRECTION('center_axis',(0.,0.,1.));
#5822=DIRECTION('ref_axis',(1.,0.,0.));
#5823=DIRECTION('center_axis',(0.,0.,1.));
#5824=DIRECTION('ref_axis',(1.,0.,0.));
#5825=DIRECTION('center_axis',(0.,0.,1.));
#5826=DIRECTION('ref_axis',(1.,0.,0.));
#5827=DIRECTION('center_axis',(0.,0.,1.));
#5828=DIRECTION('ref_axis',(1.,0.,0.));
#5829=DIRECTION('',(0.,0.,1.));
#5830=DIRECTION('center_axis',(1.,0.,0.));
#5831=DIRECTION('ref_axis',(0.,0.,-1.));
#5832=DIRECTION('center_axis',(1.,0.,0.));
#5833=DIRECTION('ref_axis',(0.,0.,-1.));
#5834=DIRECTION('',(1.,0.,0.));
#5835=DIRECTION('center_axis',(-1.,0.,0.));
#5836=DIRECTION('ref_axis',(0.,0.,-1.));
#5837=DIRECTION('center_axis',(1.,0.,0.));
#5838=DIRECTION('ref_axis',(0.,1.,0.));
#5839=DIRECTION('',(0.,-1.,0.));
#5840=DIRECTION('center_axis',(-1.,0.,0.));
#5841=DIRECTION('ref_axis',(0.,-1.,0.));
#5842=DIRECTION('',(0.,-1.,0.));
#5843=DIRECTION('center_axis',(0.,0.,1.));
#5844=DIRECTION('ref_axis',(1.,0.,0.));
#7289=CARTESIAN_POINT('',(0.,0.,0.));
#7290=CARTESIAN_POINT('Origin',(11.5,0.,7.4));
#7291=CARTESIAN_POINT('',(10.,2.2,7.4));
#7292=CARTESIAN_POINT('',(10.,-2.2,7.4));
#7293=CARTESIAN_POINT('',(10.,2.,7.4));
#7294=CARTESIAN_POINT('',(13.,-2.2,7.4));
#7295=CARTESIAN_POINT('',(10.,-2.2,7.4));
#7296=CARTESIAN_POINT('',(13.,2.2,7.4));
#7297=CARTESIAN_POINT('',(13.,-2.,7.4));
#7298=CARTESIAN_POINT('',(13.,2.2,7.4));
#7299=CARTESIAN_POINT('',(10.2,1.5,7.4));
#7300=CARTESIAN_POINT('Origin',(10.7,1.5,7.4));
#7301=CARTESIAN_POINT('',(10.2,-1.5,7.4));
#7302=CARTESIAN_POINT('Origin',(10.7,-1.5,7.4));
#7303=CARTESIAN_POINT('Origin',(13.,2.2,1.));
#7304=CARTESIAN_POINT('',(13.,2.2,1.));
#7305=CARTESIAN_POINT('',(10.,2.2,1.));
#7306=CARTESIAN_POINT('',(13.,2.2,1.));
#7307=CARTESIAN_POINT('',(10.,2.2,1.));
#7308=CARTESIAN_POINT('',(13.,2.2,7.2));
#7309=CARTESIAN_POINT('Origin',(10.,-2.2,1.));
#7310=CARTESIAN_POINT('',(10.,-2.2,1.));
#7311=CARTESIAN_POINT('',(13.,-2.2,1.));
#7312=CARTESIAN_POINT('',(10.,-2.2,1.));
#7313=CARTESIAN_POINT('',(13.,-2.2,1.));
#7314=CARTESIAN_POINT('',(10.,-2.2,7.2));
#7315=CARTESIAN_POINT('Origin',(9.9,1.2,4.05));
#7316=CARTESIAN_POINT('',(10.,1.2,4.215));
#7317=CARTESIAN_POINT('Origin',(10.,1.2,4.05));
#7318=CARTESIAN_POINT('',(10.3,1.2,4.215));
#7319=CARTESIAN_POINT('',(9.9,1.2,4.215));
#7320=CARTESIAN_POINT('',(10.2185698389174,1.365,4.05));
#7321=CARTESIAN_POINT('Ctrl Pts',(10.2185698389174,1.365,4.05));
#7322=CARTESIAN_POINT('Ctrl Pts',(10.2185698389174,1.365,4.02952043356281));
#7323=CARTESIAN_POINT('Ctrl Pts',(10.2196511820674,1.360940751691,4.00771516465356));
#7324=CARTESIAN_POINT('Ctrl Pts',(10.2246631762912,1.34467012765305,3.96777784587771));
#7325=CARTESIAN_POINT('Ctrl Pts',(10.2286736827823,1.33246344039378,3.94965394795779));
#7326=CARTESIAN_POINT('Ctrl Pts',(10.2402354326321,1.30274117773169,3.91885215023316));
#7327=CARTESIAN_POINT('Ctrl Pts',(10.2490773513426,1.28266254990227,3.90542718243916));
#7328=CARTESIAN_POINT('Ctrl Pts',(10.2717677906972,1.24080126498159,3.8885390180969));
#7329=CARTESIAN_POINT('Ctrl Pts',(10.2856850788648,1.21908656151361,3.885));
#7330=CARTESIAN_POINT('Ctrl Pts',(10.319085409969,1.17455278670803,3.885));
#7331=CARTESIAN_POINT('Ctrl Pts',(10.3419048713612,1.14954238521319,3.89106755072681));
#7332=CARTESIAN_POINT('Ctrl Pts',(10.3901989916138,1.10620312192356,3.91213177324836));
#7333=CARTESIAN_POINT('Ctrl Pts',(10.415674165106,1.08782446907905,3.92702466368572));
#7334=CARTESIAN_POINT('Ctrl Pts',(10.4559623955469,1.06313017986469,3.95639578484302));
#7335=CARTESIAN_POINT('Ctrl Pts',(10.4744285153863,1.05346991878665,3.97182573634243));
#7336=CARTESIAN_POINT('Ctrl Pts',(10.4968465722861,1.04305739521201,3.99819879372234));
#7337=CARTESIAN_POINT('Ctrl Pts',(10.5033924526994,1.04024696261202,4.00748456076932));
#7338=CARTESIAN_POINT('Ctrl Pts',(10.5130578430487,1.03623280243464,4.02744119259084));
#7339=CARTESIAN_POINT('Ctrl Pts',(10.5162202405051,1.035,4.03808539531883));
#7340=CARTESIAN_POINT('Ctrl Pts',(10.5162202405051,1.035,4.06191460468117));
#7341=CARTESIAN_POINT('Ctrl Pts',(10.5130578430487,1.03623280243464,4.07255880740916));
#7342=CARTESIAN_POINT('Ctrl Pts',(10.5033924526994,1.04024696261203,4.09251543923068));
#7343=CARTESIAN_POINT('Ctrl Pts',(10.4968465722861,1.04305739521201,4.10180120627766));
#7344=CARTESIAN_POINT('Ctrl Pts',(10.4744285153863,1.05346991878665,4.12817426365757));
#7345=CARTESIAN_POINT('Ctrl Pts',(10.4559623955469,1.06313017986469,4.14360421515698));
#7346=CARTESIAN_POINT('Ctrl Pts',(10.415674165106,1.08782446907905,4.17297533631428));
#7347=CARTESIAN_POINT('Ctrl Pts',(10.3901989916138,1.10620312192356,4.18786822675164));
#7348=CARTESIAN_POINT('Ctrl Pts',(10.3419048713612,1.14954238521319,4.20893244927319));
#7349=CARTESIAN_POINT('Ctrl Pts',(10.319085409969,1.17455278670803,4.215));
#7350=CARTESIAN_POINT('Ctrl Pts',(10.3,1.2,4.215));
#7351=CARTESIAN_POINT('Ctrl Pts',(10.3,1.2,4.215));
#7352=CARTESIAN_POINT('Ctrl Pts',(10.2856850788648,1.21908656151361,4.215));
#7353=CARTESIAN_POINT('Ctrl Pts',(10.2717677906972,1.24080126498159,4.2114609819031));
#7354=CARTESIAN_POINT('Ctrl Pts',(10.2490773513426,1.28266254990227,4.19457281756084));
#7355=CARTESIAN_POINT('Ctrl Pts',(10.2402354326322,1.30274117773169,4.18114784976684));
#7356=CARTESIAN_POINT('Ctrl Pts',(10.2286736827823,1.33246344039378,4.15034605204221));
#7357=CARTESIAN_POINT('Ctrl Pts',(10.2246631762912,1.34467012765305,4.13222215412229));
#7358=CARTESIAN_POINT('Ctrl Pts',(10.2196511820674,1.360940751691,4.09228483534644));
#7359=CARTESIAN_POINT('Ctrl Pts',(10.2185698389174,1.365,4.07047956643719));
#7360=CARTESIAN_POINT('Ctrl Pts',(10.2185698389174,1.365,4.05));
#7361=CARTESIAN_POINT('Origin',(9.9,1.2,4.05));
#7362=CARTESIAN_POINT('',(11.1814301610826,1.365,4.05));
#7363=CARTESIAN_POINT('',(11.1,1.2,4.215));
#7364=CARTESIAN_POINT('Ctrl Pts',(11.1814301610826,1.365,4.05));
#7365=CARTESIAN_POINT('Ctrl Pts',(11.1814301610826,1.365,4.07047956643719));
#7366=CARTESIAN_POINT('Ctrl Pts',(11.1803488179326,1.360940751691,4.09228483534644));
#7367=CARTESIAN_POINT('Ctrl Pts',(11.1753368237088,1.34467012765305,4.13222215412229));
#7368=CARTESIAN_POINT('Ctrl Pts',(11.1713263172177,1.33246344039378,4.15034605204221));
#7369=CARTESIAN_POINT('Ctrl Pts',(11.1597645673678,1.30274117773169,4.18114784976684));
#7370=CARTESIAN_POINT('Ctrl Pts',(11.1509226486574,1.28266254990227,4.19457281756084));
#7371=CARTESIAN_POINT('Ctrl Pts',(11.1282322093028,1.24080126498159,4.2114609819031));
#7372=CARTESIAN_POINT('Ctrl Pts',(11.1143149211352,1.21908656151361,4.215));
#7373=CARTESIAN_POINT('Ctrl Pts',(11.1,1.2,4.215));
#7374=CARTESIAN_POINT('Ctrl Pts',(11.1,1.2,4.215));
#7375=CARTESIAN_POINT('Ctrl Pts',(11.080914590031,1.17455278670802,4.215));
#7376=CARTESIAN_POINT('Ctrl Pts',(11.0580951286388,1.14954238521319,4.20893244927319));
#7377=CARTESIAN_POINT('Ctrl Pts',(11.0098010083862,1.10620312192356,4.18786822675164));
#7378=CARTESIAN_POINT('Ctrl Pts',(10.984325834894,1.08782446907905,4.17297533631428));
#7379=CARTESIAN_POINT('Ctrl Pts',(10.9440376044531,1.06313017986469,4.14360421515698));
#7380=CARTESIAN_POINT('Ctrl Pts',(10.9255714846137,1.05346991878665,4.12817426365757));
#7381=CARTESIAN_POINT('Ctrl Pts',(10.9031534277139,1.04305739521201,4.10180120627766));
#7382=CARTESIAN_POINT('Ctrl Pts',(10.8966075473006,1.04024696261203,4.09251543923068));
#7383=CARTESIAN_POINT('Ctrl Pts',(10.8869421569513,1.03623280243464,4.07255880740916));
#7384=CARTESIAN_POINT('Ctrl Pts',(10.8837797594949,1.035,4.06191460468117));
#7385=CARTESIAN_POINT('Ctrl Pts',(10.8837797594949,1.035,4.03808539531883));
#7386=CARTESIAN_POINT('Ctrl Pts',(10.8869421569513,1.03623280243464,4.02744119259084));
#7387=CARTESIAN_POINT('Ctrl Pts',(10.8966075473006,1.04024696261202,4.00748456076932));
#7388=CARTESIAN_POINT('Ctrl Pts',(10.9031534277139,1.04305739521201,3.99819879372234));
#7389=CARTESIAN_POINT('Ctrl Pts',(10.9255714846137,1.05346991878665,3.97182573634243));
#7390=CARTESIAN_POINT('Ctrl Pts',(10.9440376044531,1.06313017986469,3.95639578484302));
#7391=CARTESIAN_POINT('Ctrl Pts',(10.984325834894,1.08782446907905,3.92702466368572));
#7392=CARTESIAN_POINT('Ctrl Pts',(11.0098010083862,1.10620312192356,3.91213177324836));
#7393=CARTESIAN_POINT('Ctrl Pts',(11.0580951286388,1.14954238521319,3.89106755072681));
#7394=CARTESIAN_POINT('Ctrl Pts',(11.080914590031,1.17455278670803,3.885));
#7395=CARTESIAN_POINT('Ctrl Pts',(11.1143149211352,1.21908656151361,3.885));
#7396=CARTESIAN_POINT('Ctrl Pts',(11.1282322093028,1.24080126498159,3.8885390180969));
#7397=CARTESIAN_POINT('Ctrl Pts',(11.1509226486574,1.28266254990227,3.90542718243916));
#7398=CARTESIAN_POINT('Ctrl Pts',(11.1597645673678,1.30274117773169,3.91885215023316));
#7399=CARTESIAN_POINT('Ctrl Pts',(11.1713263172177,1.33246344039378,3.94965394795779));
#7400=CARTESIAN_POINT('Ctrl Pts',(11.1753368237088,1.34467012765305,3.96777784587771));
#7401=CARTESIAN_POINT('Ctrl Pts',(11.1803488179326,1.360940751691,4.00771516465356));
#7402=CARTESIAN_POINT('Ctrl Pts',(11.1814301610826,1.365,4.02952043356281));
#7403=CARTESIAN_POINT('Ctrl Pts',(11.1814301610826,1.365,4.05));
#7404=CARTESIAN_POINT('',(13.,1.2,4.215));
#7405=CARTESIAN_POINT('',(9.9,1.2,4.215));
#7406=CARTESIAN_POINT('Origin',(13.,1.2,4.05));
#7407=CARTESIAN_POINT('Origin',(9.9,-1.2,6.45));
#7408=CARTESIAN_POINT('',(10.,-1.2,6.615));
#7409=CARTESIAN_POINT('Origin',(10.,-1.2,6.45));
#7410=CARTESIAN_POINT('',(10.3,-1.2,6.615));
#7411=CARTESIAN_POINT('',(9.9,-1.2,6.615));
#7412=CARTESIAN_POINT('',(10.5162202405051,-1.035,6.45));
#7413=CARTESIAN_POINT('Ctrl Pts',(10.5162202405051,-1.035,6.45));
#7414=CARTESIAN_POINT('Ctrl Pts',(10.5162202405051,-1.035,6.44062045354281));
#7415=CARTESIAN_POINT('Ctrl Pts',(10.5140205633862,-1.0358566636217,6.43083371614971));
#7416=CARTESIAN_POINT('Ctrl Pts',(10.5063054900173,-1.03902296892558,6.41262650433697));
#7417=CARTESIAN_POINT('Ctrl Pts',(10.5008967482507,-1.04131297855552,6.4041576160186));
#7418=CARTESIAN_POINT('Ctrl Pts',(10.4762824962743,-1.05234965200392,6.37165968077989));
#7419=CARTESIAN_POINT('Ctrl Pts',(10.4475863157778,-1.0674330397717,6.34922172243674));
#7420=CARTESIAN_POINT('Ctrl Pts',(10.4028942700183,-1.09707700316755,6.31957775904089));
#7421=CARTESIAN_POINT('Ctrl Pts',(10.3802569440026,-1.11447899483743,6.30721461318364));
#7422=CARTESIAN_POINT('Ctrl Pts',(10.3373328915009,-1.15455153425976,6.28988771813691));
#7423=CARTESIAN_POINT('Ctrl Pts',(10.3170531808664,-1.17726242551144,6.285));
#7424=CARTESIAN_POINT('Ctrl Pts',(10.2859943020946,-1.21867426387382,6.285));
#7425=CARTESIAN_POINT('Ctrl Pts',(10.2723294055107,-1.2399125795835,6.28838530514966));
#7426=CARTESIAN_POINT('Ctrl Pts',(10.249906982231,-1.28099344112303,6.30456138651949));
#7427=CARTESIAN_POINT('Ctrl Pts',(10.2410876841917,-1.30077258467692,6.31742734688536));
#7428=CARTESIAN_POINT('Ctrl Pts',(10.2291861979204,-1.33097165226366,6.3476264144721));
#7429=CARTESIAN_POINT('Ctrl Pts',(10.2249675898062,-1.34371971020651,6.36599964223317));
#7430=CARTESIAN_POINT('Ctrl Pts',(10.2197033363378,-1.36073611264639,6.40669500858237));
#7431=CARTESIAN_POINT('Ctrl Pts',(10.2185698389174,-1.365,6.42900759846042));
#7432=CARTESIAN_POINT('Ctrl Pts',(10.2185698389174,-1.365,6.47047956643719));
#7433=CARTESIAN_POINT('Ctrl Pts',(10.2196511820674,-1.360940751691,6.49228483534644));
#7434=CARTESIAN_POINT('Ctrl Pts',(10.2246631762912,-1.34467012765305,6.53222215412229));
#7435=CARTESIAN_POINT('Ctrl Pts',(10.2286736827823,-1.33246344039378,6.55034605204221));
#7436=CARTESIAN_POINT('Ctrl Pts',(10.2402354326322,-1.30274117773169,6.58114784976684));
#7437=CARTESIAN_POINT('Ctrl Pts',(10.2490773513426,-1.28266254990227,6.59457281756084));
#7438=CARTESIAN_POINT('Ctrl Pts',(10.2717677906972,-1.24080126498159,6.6114609819031));
#7439=CARTESIAN_POINT('Ctrl Pts',(10.2856850788648,-1.21908656151361,6.615));
#7440=CARTESIAN_POINT('Ctrl Pts',(10.3,-1.2,6.615));
#7441=CARTESIAN_POINT('Ctrl Pts',(10.3,-1.2,6.615));
#7442=CARTESIAN_POINT('Ctrl Pts',(10.319085409969,-1.17455278670802,6.615));
#7443=CARTESIAN_POINT('Ctrl Pts',(10.3419048713612,-1.14954238521319,6.60893244927319));
#7444=CARTESIAN_POINT('Ctrl Pts',(10.3901989916138,-1.10620312192356,6.58786822675164));
#7445=CARTESIAN_POINT('Ctrl Pts',(10.415674165106,-1.08782446907905,6.57297533631428));
#7446=CARTESIAN_POINT('Ctrl Pts',(10.4559623955469,-1.06313017986469,6.54360421515698));
#7447=CARTESIAN_POINT('Ctrl Pts',(10.4744285153863,-1.05346991878665,6.52817426365758));
#7448=CARTESIAN_POINT('Ctrl Pts',(10.4968465722861,-1.04305739521201,6.50180120627766));
#7449=CARTESIAN_POINT('Ctrl Pts',(10.5033924526994,-1.04024696261203,6.49251543923068));
#7450=CARTESIAN_POINT('Ctrl Pts',(10.5130578430487,-1.03623280243464,6.47255880740916));
#7451=CARTESIAN_POINT('Ctrl Pts',(10.5162202405051,-1.035,6.46191460468117));
#7452=CARTESIAN_POINT('Ctrl Pts',(10.5162202405051,-1.035,6.45));
#7453=CARTESIAN_POINT('Origin',(9.9,-1.2,6.45));
#7454=CARTESIAN_POINT('',(10.8837797594949,-1.035,6.45));
#7455=CARTESIAN_POINT('',(11.1,-1.2,6.615));
#7456=CARTESIAN_POINT('Ctrl Pts',(10.8837797594949,-1.035,6.45));
#7457=CARTESIAN_POINT('Ctrl Pts',(10.8837797594949,-1.035,6.46191460468117));
#7458=CARTESIAN_POINT('Ctrl Pts',(10.8869421569513,-1.03623280243464,6.47255880740916));
#7459=CARTESIAN_POINT('Ctrl Pts',(10.8966075473006,-1.04024696261203,6.49251543923068));
#7460=CARTESIAN_POINT('Ctrl Pts',(10.9031534277139,-1.04305739521201,6.50180120627766));
#7461=CARTESIAN_POINT('Ctrl Pts',(10.9255714846137,-1.05346991878665,6.52817426365758));
#7462=CARTESIAN_POINT('Ctrl Pts',(10.9440376044531,-1.06313017986469,6.54360421515698));
#7463=CARTESIAN_POINT('Ctrl Pts',(10.984325834894,-1.08782446907905,6.57297533631428));
#7464=CARTESIAN_POINT('Ctrl Pts',(11.0098010083862,-1.10620312192356,6.58786822675164));
#7465=CARTESIAN_POINT('Ctrl Pts',(11.0580951286388,-1.14954238521319,6.60893244927319));
#7466=CARTESIAN_POINT('Ctrl Pts',(11.080914590031,-1.17455278670802,6.615));
#7467=CARTESIAN_POINT('Ctrl Pts',(11.1,-1.2,6.615));
#7468=CARTESIAN_POINT('Ctrl Pts',(11.1,-1.2,6.615));
#7469=CARTESIAN_POINT('Ctrl Pts',(11.1143149211352,-1.21908656151361,6.615));
#7470=CARTESIAN_POINT('Ctrl Pts',(11.1282322093028,-1.24080126498159,6.6114609819031));
#7471=CARTESIAN_POINT('Ctrl Pts',(11.1509226486574,-1.28266254990227,6.59457281756084));
#7472=CARTESIAN_POINT('Ctrl Pts',(11.1597645673678,-1.30274117773169,6.58114784976684));
#7473=CARTESIAN_POINT('Ctrl Pts',(11.1713263172177,-1.33246344039378,6.55034605204221));
#7474=CARTESIAN_POINT('Ctrl Pts',(11.1753368237088,-1.34467012765305,6.53222215412229));
#7475=CARTESIAN_POINT('Ctrl Pts',(11.1803488179326,-1.360940751691,6.49228483534644));
#7476=CARTESIAN_POINT('Ctrl Pts',(11.1814301610826,-1.365,6.47047956643719));
#7477=CARTESIAN_POINT('Ctrl Pts',(11.1814301610826,-1.365,6.42900759846042));
#7478=CARTESIAN_POINT('Ctrl Pts',(11.1802966636622,-1.36073611264639,6.40669500858237));
#7479=CARTESIAN_POINT('Ctrl Pts',(11.1750324101937,-1.34371971020651,6.36599964223317));
#7480=CARTESIAN_POINT('Ctrl Pts',(11.1708138020796,-1.33097165226366,6.3476264144721));
#7481=CARTESIAN_POINT('Ctrl Pts',(11.1589123158083,-1.30077258467692,6.31742734688536));
#7482=CARTESIAN_POINT('Ctrl Pts',(11.150093017769,-1.28099344112303,6.30456138651949));
#7483=CARTESIAN_POINT('Ctrl Pts',(11.1276705944893,-1.23991257958351,6.28838530514966));
#7484=CARTESIAN_POINT('Ctrl Pts',(11.1140056979054,-1.21867426387382,6.285));
#7485=CARTESIAN_POINT('Ctrl Pts',(11.0829468191336,-1.17726242551144,6.285));
#7486=CARTESIAN_POINT('Ctrl Pts',(11.0626671084991,-1.15455153425976,6.28988771813691));
#7487=CARTESIAN_POINT('Ctrl Pts',(11.0197430559974,-1.11447899483743,6.30721461318364));
#7488=CARTESIAN_POINT('Ctrl Pts',(10.9971057299817,-1.09707700316755,6.31957775904089));
#7489=CARTESIAN_POINT('Ctrl Pts',(10.9524136842222,-1.0674330397717,6.34922172243674));
#7490=CARTESIAN_POINT('Ctrl Pts',(10.9237175037257,-1.05234965200392,6.37165968077989));
#7491=CARTESIAN_POINT('Ctrl Pts',(10.8991032517493,-1.04131297855552,6.4041576160186));
#7492=CARTESIAN_POINT('Ctrl Pts',(10.8936945099827,-1.03902296892558,6.41262650433697));
#7493=CARTESIAN_POINT('Ctrl Pts',(10.8859794366138,-1.0358566636217,6.43083371614971));
#7494=CARTESIAN_POINT('Ctrl Pts',(10.8837797594949,-1.035,6.44062045354281));
#7495=CARTESIAN_POINT('Ctrl Pts',(10.8837797594949,-1.035,6.45));
#7496=CARTESIAN_POINT('',(13.,-1.2,6.615));
#7497=CARTESIAN_POINT('',(9.9,-1.2,6.615));
#7498=CARTESIAN_POINT('Origin',(13.,-1.2,6.45));
#7499=CARTESIAN_POINT('Origin',(9.9,-1.2,4.05));
#7500=CARTESIAN_POINT('',(10.,-1.2,4.215));
#7501=CARTESIAN_POINT('Origin',(10.,-1.2,4.05));
#7502=CARTESIAN_POINT('',(10.3,-1.2,4.215));
#7503=CARTESIAN_POINT('',(9.9,-1.2,4.215));
#7504=CARTESIAN_POINT('',(10.5162202405051,-1.035,4.05));
#7505=CARTESIAN_POINT('Ctrl Pts',(10.5162202405051,-1.035,4.05));
#7506=CARTESIAN_POINT('Ctrl Pts',(10.5162202405051,-1.035,4.03808539531883));
#7507=CARTESIAN_POINT('Ctrl Pts',(10.5130578430487,-1.03623280243464,4.02744119259084));
#7508=CARTESIAN_POINT('Ctrl Pts',(10.5033924526994,-1.04024696261202,4.00748456076932));
#7509=CARTESIAN_POINT('Ctrl Pts',(10.4968465722861,-1.04305739521201,3.99819879372234));
#7510=CARTESIAN_POINT('Ctrl Pts',(10.4744285153863,-1.05346991878665,3.97182573634243));
#7511=CARTESIAN_POINT('Ctrl Pts',(10.4559623955469,-1.06313017986469,3.95639578484302));
#7512=CARTESIAN_POINT('Ctrl Pts',(10.415674165106,-1.08782446907905,3.92702466368572));
#7513=CARTESIAN_POINT('Ctrl Pts',(10.3901989916138,-1.10620312192356,3.91213177324836));
#7514=CARTESIAN_POINT('Ctrl Pts',(10.3419048713612,-1.14954238521319,3.89106755072681));
#7515=CARTESIAN_POINT('Ctrl Pts',(10.319085409969,-1.17455278670803,3.885));
#7516=CARTESIAN_POINT('Ctrl Pts',(10.2856850788648,-1.21908656151361,3.885));
#7517=CARTESIAN_POINT('Ctrl Pts',(10.2717677906972,-1.24080126498159,3.88853901809689));
#7518=CARTESIAN_POINT('Ctrl Pts',(10.2490773513426,-1.28266254990227,3.90542718243916));
#7519=CARTESIAN_POINT('Ctrl Pts',(10.2402354326321,-1.30274117773169,3.91885215023316));
#7520=CARTESIAN_POINT('Ctrl Pts',(10.2286736827823,-1.33246344039378,3.94965394795779));
#7521=CARTESIAN_POINT('Ctrl Pts',(10.2246631762912,-1.34467012765305,3.96777784587771));
#7522=CARTESIAN_POINT('Ctrl Pts',(10.2196511820674,-1.360940751691,4.00771516465356));
#7523=CARTESIAN_POINT('Ctrl Pts',(10.2185698389174,-1.365,4.02952043356281));
#7524=CARTESIAN_POINT('Ctrl Pts',(10.2185698389174,-1.365,4.07047956643719));
#7525=CARTESIAN_POINT('Ctrl Pts',(10.2196511820674,-1.360940751691,4.09228483534644));
#7526=CARTESIAN_POINT('Ctrl Pts',(10.2246631762912,-1.34467012765305,4.13222215412229));
#7527=CARTESIAN_POINT('Ctrl Pts',(10.2286736827823,-1.33246344039378,4.15034605204221));
#7528=CARTESIAN_POINT('Ctrl Pts',(10.2402354326321,-1.30274117773169,4.18114784976684));
#7529=CARTESIAN_POINT('Ctrl Pts',(10.2490773513426,-1.28266254990227,4.19457281756084));
#7530=CARTESIAN_POINT('Ctrl Pts',(10.2717677906972,-1.24080126498159,4.2114609819031));
#7531=CARTESIAN_POINT('Ctrl Pts',(10.2856850788648,-1.21908656151361,4.215));
#7532=CARTESIAN_POINT('Ctrl Pts',(10.3,-1.2,4.215));
#7533=CARTESIAN_POINT('Ctrl Pts',(10.3,-1.2,4.215));
#7534=CARTESIAN_POINT('Ctrl Pts',(10.319085409969,-1.17455278670802,4.215));
#7535=CARTESIAN_POINT('Ctrl Pts',(10.3419048713612,-1.14954238521319,4.20893244927319));
#7536=CARTESIAN_POINT('Ctrl Pts',(10.3901989916138,-1.10620312192356,4.18786822675164));
#7537=CARTESIAN_POINT('Ctrl Pts',(10.415674165106,-1.08782446907905,4.17297533631428));
#7538=CARTESIAN_POINT('Ctrl Pts',(10.4559623955469,-1.06313017986469,4.14360421515698));
#7539=CARTESIAN_POINT('Ctrl Pts',(10.4744285153863,-1.05346991878665,4.12817426365757));
#7540=CARTESIAN_POINT('Ctrl Pts',(10.4968465722861,-1.04305739521201,4.10180120627766));
#7541=CARTESIAN_POINT('Ctrl Pts',(10.5033924526994,-1.04024696261203,4.09251543923068));
#7542=CARTESIAN_POINT('Ctrl Pts',(10.5130578430487,-1.03623280243464,4.07255880740916));
#7543=CARTESIAN_POINT('Ctrl Pts',(10.5162202405051,-1.035,4.06191460468117));
#7544=CARTESIAN_POINT('Ctrl Pts',(10.5162202405051,-1.035,4.05));
#7545=CARTESIAN_POINT('Origin',(9.9,-1.2,4.05));
#7546=CARTESIAN_POINT('',(10.8837797594949,-1.035,4.05));
#7547=CARTESIAN_POINT('',(11.1,-1.2,4.215));
#7548=CARTESIAN_POINT('Ctrl Pts',(10.8837797594949,-1.035,4.05));
#7549=CARTESIAN_POINT('Ctrl Pts',(10.8837797594949,-1.035,4.06191460468117));
#7550=CARTESIAN_POINT('Ctrl Pts',(10.8869421569513,-1.03623280243464,4.07255880740916));
#7551=CARTESIAN_POINT('Ctrl Pts',(10.8966075473006,-1.04024696261203,4.09251543923068));
#7552=CARTESIAN_POINT('Ctrl Pts',(10.9031534277139,-1.04305739521201,4.10180120627766));
#7553=CARTESIAN_POINT('Ctrl Pts',(10.9255714846137,-1.05346991878665,4.12817426365757));
#7554=CARTESIAN_POINT('Ctrl Pts',(10.9440376044531,-1.06313017986469,4.14360421515698));
#7555=CARTESIAN_POINT('Ctrl Pts',(10.984325834894,-1.08782446907905,4.17297533631428));
#7556=CARTESIAN_POINT('Ctrl Pts',(11.0098010083862,-1.10620312192355,4.18786822675163));
#7557=CARTESIAN_POINT('Ctrl Pts',(11.0580951286388,-1.14954238521319,4.20893244927319));
#7558=CARTESIAN_POINT('Ctrl Pts',(11.080914590031,-1.17455278670803,4.215));
#7559=CARTESIAN_POINT('Ctrl Pts',(11.1,-1.2,4.215));
#7560=CARTESIAN_POINT('Ctrl Pts',(11.1,-1.2,4.215));
#7561=CARTESIAN_POINT('Ctrl Pts',(11.1143149211352,-1.21908656151361,4.215));
#7562=CARTESIAN_POINT('Ctrl Pts',(11.1282322093028,-1.24080126498159,4.2114609819031));
#7563=CARTESIAN_POINT('Ctrl Pts',(11.1509226486574,-1.28266254990227,4.19457281756084));
#7564=CARTESIAN_POINT('Ctrl Pts',(11.1597645673678,-1.30274117773169,4.18114784976684));
#7565=CARTESIAN_POINT('Ctrl Pts',(11.1713263172177,-1.33246344039378,4.15034605204221));
#7566=CARTESIAN_POINT('Ctrl Pts',(11.1753368237088,-1.34467012765305,4.13222215412229));
#7567=CARTESIAN_POINT('Ctrl Pts',(11.1803488179326,-1.360940751691,4.09228483534644));
#7568=CARTESIAN_POINT('Ctrl Pts',(11.1814301610826,-1.365,4.07047956643719));
#7569=CARTESIAN_POINT('Ctrl Pts',(11.1814301610826,-1.365,4.02952043356281));
#7570=CARTESIAN_POINT('Ctrl Pts',(11.1803488179326,-1.360940751691,4.00771516465356));
#7571=CARTESIAN_POINT('Ctrl Pts',(11.1753368237088,-1.34467012765305,3.96777784587771));
#7572=CARTESIAN_POINT('Ctrl Pts',(11.1713263172177,-1.33246344039378,3.94965394795779));
#7573=CARTESIAN_POINT('Ctrl Pts',(11.1597645673678,-1.30274117773169,3.91885215023316));
#7574=CARTESIAN_POINT('Ctrl Pts',(11.1509226486574,-1.28266254990227,3.90542718243916));
#7575=CARTESIAN_POINT('Ctrl Pts',(11.1282322093028,-1.24080126498159,3.8885390180969));
#7576=CARTESIAN_POINT('Ctrl Pts',(11.1143149211352,-1.21908656151361,3.885));
#7577=CARTESIAN_POINT('Ctrl Pts',(11.080914590031,-1.17455278670803,3.885));
#7578=CARTESIAN_POINT('Ctrl Pts',(11.0580951286388,-1.14954238521319,3.89106755072681));
#7579=CARTESIAN_POINT('Ctrl Pts',(11.0098010083862,-1.10620312192356,3.91213177324836));
#7580=CARTESIAN_POINT('Ctrl Pts',(10.984325834894,-1.08782446907905,3.92702466368572));
#7581=CARTESIAN_POINT('Ctrl Pts',(10.9440376044531,-1.06313017986469,3.95639578484302));
#7582=CARTESIAN_POINT('Ctrl Pts',(10.9255714846137,-1.05346991878665,3.97182573634243));
#7583=CARTESIAN_POINT('Ctrl Pts',(10.9031534277139,-1.04305739521201,3.99819879372234));
#7584=CARTESIAN_POINT('Ctrl Pts',(10.8966075473006,-1.04024696261202,4.00748456076932));
#7585=CARTESIAN_POINT('Ctrl Pts',(10.8869421569513,-1.03623280243464,4.02744119259084));
#7586=CARTESIAN_POINT('Ctrl Pts',(10.8837797594949,-1.035,4.03808539531883));
#7587=CARTESIAN_POINT('Ctrl Pts',(10.8837797594949,-1.035,4.05));
#7588=CARTESIAN_POINT('',(13.,-1.2,4.215));
#7589=CARTESIAN_POINT('',(9.9,-1.2,4.215));
#7590=CARTESIAN_POINT('Origin',(13.,-1.2,4.05));
#7591=CARTESIAN_POINT('Origin',(9.9,1.2,6.45));
#7592=CARTESIAN_POINT('',(10.,1.2,6.615));
#7593=CARTESIAN_POINT('Origin',(10.,1.2,6.45));
#7594=CARTESIAN_POINT('',(10.3,1.2,6.615));
#7595=CARTESIAN_POINT('',(9.9,1.2,6.615));
#7596=CARTESIAN_POINT('',(10.2185698389174,1.365,6.45));
#7597=CARTESIAN_POINT('Ctrl Pts',(10.2185698389174,1.365,6.45));
#7598=CARTESIAN_POINT('Ctrl Pts',(10.2185698389174,1.365,6.42900759846042));
#7599=CARTESIAN_POINT('Ctrl Pts',(10.2197033363378,1.36073611264639,6.40669500858237));
#7600=CARTESIAN_POINT('Ctrl Pts',(10.2249675898062,1.34371971020651,6.36599964223317));
#7601=CARTESIAN_POINT('Ctrl Pts',(10.2291861979204,1.33097165226366,6.3476264144721));
#7602=CARTESIAN_POINT('Ctrl Pts',(10.2410876841917,1.30077258467692,6.31742734688536));
#7603=CARTESIAN_POINT('Ctrl Pts',(10.249906982231,1.28099344112303,6.30456138651949));
#7604=CARTESIAN_POINT('Ctrl Pts',(10.2723294055107,1.2399125795835,6.28838530514966));
#7605=CARTESIAN_POINT('Ctrl Pts',(10.2859943020946,1.21867426387382,6.285));
#7606=CARTESIAN_POINT('Ctrl Pts',(10.3170531808664,1.17726242551144,6.285));
#7607=CARTESIAN_POINT('Ctrl Pts',(10.3373328915009,1.15455153425976,6.28988771813691));
#7608=CARTESIAN_POINT('Ctrl Pts',(10.3802569440026,1.11447899483743,6.30721461318364));
#7609=CARTESIAN_POINT('Ctrl Pts',(10.4028942700183,1.09707700316755,6.31957775904089));
#7610=CARTESIAN_POINT('Ctrl Pts',(10.4475863157778,1.0674330397717,6.34922172243674));
#7611=CARTESIAN_POINT('Ctrl Pts',(10.4762824962743,1.05234965200392,6.37165968077989));
#7612=CARTESIAN_POINT('Ctrl Pts',(10.5008967482507,1.04131297855552,6.4041576160186));
#7613=CARTESIAN_POINT('Ctrl Pts',(10.5063054900173,1.03902296892558,6.41262650433697));
#7614=CARTESIAN_POINT('Ctrl Pts',(10.5140205633862,1.0358566636217,6.43083371614971));
#7615=CARTESIAN_POINT('Ctrl Pts',(10.5162202405051,1.035,6.44062045354281));
#7616=CARTESIAN_POINT('Ctrl Pts',(10.5162202405051,1.035,6.46191460468117));
#7617=CARTESIAN_POINT('Ctrl Pts',(10.5130578430487,1.03623280243464,6.47255880740916));
#7618=CARTESIAN_POINT('Ctrl Pts',(10.5033924526994,1.04024696261203,6.49251543923068));
#7619=CARTESIAN_POINT('Ctrl Pts',(10.4968465722861,1.04305739521201,6.50180120627766));
#7620=CARTESIAN_POINT('Ctrl Pts',(10.4744285153863,1.05346991878665,6.52817426365758));
#7621=CARTESIAN_POINT('Ctrl Pts',(10.4559623955469,1.06313017986469,6.54360421515698));
#7622=CARTESIAN_POINT('Ctrl Pts',(10.415674165106,1.08782446907905,6.57297533631428));
#7623=CARTESIAN_POINT('Ctrl Pts',(10.3901989916138,1.10620312192356,6.58786822675164));
#7624=CARTESIAN_POINT('Ctrl Pts',(10.3419048713612,1.14954238521319,6.60893244927319));
#7625=CARTESIAN_POINT('Ctrl Pts',(10.319085409969,1.17455278670802,6.615));
#7626=CARTESIAN_POINT('Ctrl Pts',(10.3,1.2,6.615));
#7627=CARTESIAN_POINT('Ctrl Pts',(10.3,1.2,6.615));
#7628=CARTESIAN_POINT('Ctrl Pts',(10.2856850788648,1.21908656151361,6.615));
#7629=CARTESIAN_POINT('Ctrl Pts',(10.2717677906972,1.24080126498159,6.6114609819031));
#7630=CARTESIAN_POINT('Ctrl Pts',(10.2490773513426,1.28266254990227,6.59457281756084));
#7631=CARTESIAN_POINT('Ctrl Pts',(10.2402354326321,1.30274117773169,6.58114784976684));
#7632=CARTESIAN_POINT('Ctrl Pts',(10.2286736827823,1.33246344039378,6.55034605204221));
#7633=CARTESIAN_POINT('Ctrl Pts',(10.2246631762912,1.34467012765305,6.53222215412229));
#7634=CARTESIAN_POINT('Ctrl Pts',(10.2196511820674,1.360940751691,6.49228483534644));
#7635=CARTESIAN_POINT('Ctrl Pts',(10.2185698389174,1.365,6.47047956643719));
#7636=CARTESIAN_POINT('Ctrl Pts',(10.2185698389174,1.365,6.45));
#7637=CARTESIAN_POINT('Origin',(9.9,1.2,6.45));
#7638=CARTESIAN_POINT('',(11.1814301610826,1.365,6.45));
#7639=CARTESIAN_POINT('',(11.1,1.2,6.615));
#7640=CARTESIAN_POINT('Ctrl Pts',(11.1814301610826,1.365,6.45));
#7641=CARTESIAN_POINT('Ctrl Pts',(11.1814301610826,1.365,6.47047956643719));
#7642=CARTESIAN_POINT('Ctrl Pts',(11.1803488179326,1.360940751691,6.49228483534644));
#7643=CARTESIAN_POINT('Ctrl Pts',(11.1753368237088,1.34467012765305,6.53222215412229));
#7644=CARTESIAN_POINT('Ctrl Pts',(11.1713263172177,1.33246344039378,6.55034605204221));
#7645=CARTESIAN_POINT('Ctrl Pts',(11.1597645673678,1.30274117773169,6.58114784976684));
#7646=CARTESIAN_POINT('Ctrl Pts',(11.1509226486574,1.28266254990227,6.59457281756084));
#7647=CARTESIAN_POINT('Ctrl Pts',(11.1282322093028,1.24080126498159,6.6114609819031));
#7648=CARTESIAN_POINT('Ctrl Pts',(11.1143149211352,1.21908656151361,6.615));
#7649=CARTESIAN_POINT('Ctrl Pts',(11.1,1.2,6.615));
#7650=CARTESIAN_POINT('Ctrl Pts',(11.1,1.2,6.615));
#7651=CARTESIAN_POINT('Ctrl Pts',(11.080914590031,1.17455278670803,6.615));
#7652=CARTESIAN_POINT('Ctrl Pts',(11.0580951286388,1.14954238521319,6.60893244927319));
#7653=CARTESIAN_POINT('Ctrl Pts',(11.0098010083862,1.10620312192356,6.58786822675164));
#7654=CARTESIAN_POINT('Ctrl Pts',(10.984325834894,1.08782446907905,6.57297533631428));
#7655=CARTESIAN_POINT('Ctrl Pts',(10.9440376044531,1.06313017986469,6.54360421515698));
#7656=CARTESIAN_POINT('Ctrl Pts',(10.9255714846137,1.05346991878665,6.52817426365758));
#7657=CARTESIAN_POINT('Ctrl Pts',(10.9031534277139,1.04305739521201,6.50180120627766));
#7658=CARTESIAN_POINT('Ctrl Pts',(10.8966075473006,1.04024696261203,6.49251543923068));
#7659=CARTESIAN_POINT('Ctrl Pts',(10.8869421569513,1.03623280243464,6.47255880740916));
#7660=CARTESIAN_POINT('Ctrl Pts',(10.8837797594949,1.035,6.46191460468117));
#7661=CARTESIAN_POINT('Ctrl Pts',(10.8837797594949,1.035,6.44062045354281));
#7662=CARTESIAN_POINT('Ctrl Pts',(10.8859794366138,1.0358566636217,6.43083371614971));
#7663=CARTESIAN_POINT('Ctrl Pts',(10.8936945099827,1.03902296892558,6.41262650433697));
#7664=CARTESIAN_POINT('Ctrl Pts',(10.8991032517493,1.04131297855552,6.4041576160186));
#7665=CARTESIAN_POINT('Ctrl Pts',(10.9237175037257,1.05234965200392,6.37165968077989));
#7666=CARTESIAN_POINT('Ctrl Pts',(10.9524136842222,1.0674330397717,6.34922172243674));
#7667=CARTESIAN_POINT('Ctrl Pts',(10.9971057299817,1.09707700316755,6.31957775904089));
#7668=CARTESIAN_POINT('Ctrl Pts',(11.0197430559974,1.11447899483743,6.30721461318364));
#7669=CARTESIAN_POINT('Ctrl Pts',(11.0626671084991,1.15455153425976,6.28988771813691));
#7670=CARTESIAN_POINT('Ctrl Pts',(11.0829468191336,1.17726242551144,6.285));
#7671=CARTESIAN_POINT('Ctrl Pts',(11.1140056979054,1.21867426387382,6.285));
#7672=CARTESIAN_POINT('Ctrl Pts',(11.1276705944893,1.2399125795835,6.28838530514966));
#7673=CARTESIAN_POINT('Ctrl Pts',(11.150093017769,1.28099344112303,6.30456138651949));
#7674=CARTESIAN_POINT('Ctrl Pts',(11.1589123158083,1.30077258467692,6.31742734688536));
#7675=CARTESIAN_POINT('Ctrl Pts',(11.1708138020796,1.33097165226366,6.3476264144721));
#7676=CARTESIAN_POINT('Ctrl Pts',(11.1750324101937,1.34371971020651,6.36599964223317));
#7677=CARTESIAN_POINT('Ctrl Pts',(11.1802966636622,1.36073611264639,6.40669500858237));
#7678=CARTESIAN_POINT('Ctrl Pts',(11.1814301610826,1.365,6.42900759846042));
#7679=CARTESIAN_POINT('Ctrl Pts',(11.1814301610826,1.365,6.45));
#7680=CARTESIAN_POINT('',(13.,1.2,6.615));
#7681=CARTESIAN_POINT('',(9.9,1.2,6.615));
#7682=CARTESIAN_POINT('Origin',(13.,1.2,6.45));
#7683=CARTESIAN_POINT('Origin',(10.7,1.5,2.));
#7684=CARTESIAN_POINT('',(10.2,1.5,2.));
#7685=CARTESIAN_POINT('Origin',(10.7,1.5,2.));
#7686=CARTESIAN_POINT('',(10.2,1.5,2.));
#7687=CARTESIAN_POINT('',(10.917944947177,1.05,5.25));
#7688=CARTESIAN_POINT('Ctrl Pts',(10.917944947177,1.05,5.25));
#7689=CARTESIAN_POINT('Ctrl Pts',(10.917944947177,1.05,5.19751752176563));
#7690=CARTESIAN_POINT('Ctrl Pts',(10.9096209325494,1.04560657967159,5.14124876244566));
#7691=CARTESIAN_POINT('Ctrl Pts',(10.8813992178595,1.0339550375075,5.06535990747913));
#7692=CARTESIAN_POINT('Ctrl Pts',(10.8694149146398,1.02931935924876,5.04147273982077));
#7693=CARTESIAN_POINT('Ctrl Pts',(10.839847070119,1.01970376154596,4.99863134755478));
#7694=CARTESIAN_POINT('Ctrl Pts',(10.8223106862062,1.01472209320273,4.9796449878867));
#7695=CARTESIAN_POINT('Ctrl Pts',(10.7875957538804,1.00753000589576,4.954205579358));
#7696=CARTESIAN_POINT('Ctrl Pts',(10.7711257791067,1.0047701664708,4.9450775807219));
#7697=CARTESIAN_POINT('Ctrl Pts',(10.7360319592806,1.0009878010724,4.9328814434269));
#7698=CARTESIAN_POINT('Ctrl Pts',(10.7173937944281,1.,4.92984378812836));
#7699=CARTESIAN_POINT('Ctrl Pts',(10.6826062055719,1.,4.92984378812836));
#7700=CARTESIAN_POINT('Ctrl Pts',(10.6639680407194,1.0009878010724,4.9328814434269));
#7701=CARTESIAN_POINT('Ctrl Pts',(10.6288742208933,1.0047701664708,4.9450775807219));
#7702=CARTESIAN_POINT('Ctrl Pts',(10.6124042461196,1.00753000589576,4.954205579358));
#7703=CARTESIAN_POINT('Ctrl Pts',(10.5776893137938,1.01472209320273,4.9796449878867));
#7704=CARTESIAN_POINT('Ctrl Pts',(10.560152929881,1.01970376154596,4.99863134755478));
#7705=CARTESIAN_POINT('Ctrl Pts',(10.5305850853602,1.02931935924876,5.04147273982077));
#7706=CARTESIAN_POINT('Ctrl Pts',(10.5186007821405,1.0339550375075,5.06535990747913));
#7707=CARTESIAN_POINT('Ctrl Pts',(10.4903790674506,1.04560657967159,5.14124876244566));
#7708=CARTESIAN_POINT('Ctrl Pts',(10.482055052823,1.05,5.19751752176563));
#7709=CARTESIAN_POINT('Ctrl Pts',(10.482055052823,1.05,5.30248247823437));
#7710=CARTESIAN_POINT('Ctrl Pts',(10.4903790674506,1.04560657967159,5.35875123755434));
#7711=CARTESIAN_POINT('Ctrl Pts',(10.5186007821405,1.0339550375075,5.43464009252087));
#7712=CARTESIAN_POINT('Ctrl Pts',(10.5305850853602,1.02931935924876,5.45852726017924));
#7713=CARTESIAN_POINT('Ctrl Pts',(10.560152929881,1.01970376154596,5.50136865244522));
#7714=CARTESIAN_POINT('Ctrl Pts',(10.5776893137938,1.01472209320273,5.5203550121133));
#7715=CARTESIAN_POINT('Ctrl Pts',(10.6124042461196,1.00753000589576,5.545794420642));
#7716=CARTESIAN_POINT('Ctrl Pts',(10.6288742208933,1.0047701664708,5.5549224192781));
#7717=CARTESIAN_POINT('Ctrl Pts',(10.6639680407194,1.0009878010724,5.5671185565731));
#7718=CARTESIAN_POINT('Ctrl Pts',(10.6826062055719,1.,5.57015621187164));
#7719=CARTESIAN_POINT('Ctrl Pts',(10.7173937944281,1.,5.57015621187164));
#7720=CARTESIAN_POINT('Ctrl Pts',(10.7360319592806,1.0009878010724,5.5671185565731));
#7721=CARTESIAN_POINT('Ctrl Pts',(10.7711257791067,1.0047701664708,5.5549224192781));
#7722=CARTESIAN_POINT('Ctrl Pts',(10.7875957538804,1.00753000589576,5.545794420642));
#7723=CARTESIAN_POINT('Ctrl Pts',(10.8223106862062,1.01472209320273,5.5203550121133));
#7724=CARTESIAN_POINT('Ctrl Pts',(10.839847070119,1.01970376154596,5.50136865244522));
#7725=CARTESIAN_POINT('Ctrl Pts',(10.8694149146398,1.02931935924876,5.45852726017924));
#7726=CARTESIAN_POINT('Ctrl Pts',(10.8813992178595,1.0339550375075,5.43464009252087));
#7727=CARTESIAN_POINT('Ctrl Pts',(10.9096209325494,1.04560657967159,5.35875123755434));
#7728=CARTESIAN_POINT('Ctrl Pts',(10.917944947177,1.05,5.30248247823437));
#7729=CARTESIAN_POINT('Ctrl Pts',(10.917944947177,1.05,5.25));
#7730=CARTESIAN_POINT('Origin',(10.7,1.5,2.));
#7731=CARTESIAN_POINT('',(10.425,1.5,2.));
#7732=CARTESIAN_POINT('Origin',(10.7,1.5,2.));
#7733=CARTESIAN_POINT('Origin',(10.7,1.5,0.9));
#7734=CARTESIAN_POINT('',(10.425,1.5,1.));
#7735=CARTESIAN_POINT('Origin',(10.7,1.5,1.));
#7736=CARTESIAN_POINT('',(10.425,1.5,0.9));
#7737=CARTESIAN_POINT('Origin',(10.7,-1.5,2.));
#7738=CARTESIAN_POINT('',(10.2,-1.5,2.));
#7739=CARTESIAN_POINT('Origin',(10.7,-1.5,2.));
#7740=CARTESIAN_POINT('',(10.2,-1.5,2.));
#7741=CARTESIAN_POINT('',(10.482055052823,-1.05,5.25));
#7742=CARTESIAN_POINT('Ctrl Pts',(10.482055052823,-1.05,5.25));
#7743=CARTESIAN_POINT('Ctrl Pts',(10.482055052823,-1.05,5.19751752176563));
#7744=CARTESIAN_POINT('Ctrl Pts',(10.4903790674506,-1.04560657967159,5.14124876244566));
#7745=CARTESIAN_POINT('Ctrl Pts',(10.5186007821405,-1.0339550375075,5.06535990747913));
#7746=CARTESIAN_POINT('Ctrl Pts',(10.5305850853602,-1.02931935924876,5.04147273982077));
#7747=CARTESIAN_POINT('Ctrl Pts',(10.560152929881,-1.01970376154596,4.99863134755478));
#7748=CARTESIAN_POINT('Ctrl Pts',(10.5776893137938,-1.01472209320273,4.9796449878867));
#7749=CARTESIAN_POINT('Ctrl Pts',(10.6124042461196,-1.00753000589576,4.954205579358));
#7750=CARTESIAN_POINT('Ctrl Pts',(10.6288742208933,-1.0047701664708,4.9450775807219));
#7751=CARTESIAN_POINT('Ctrl Pts',(10.6639680407194,-1.0009878010724,4.9328814434269));
#7752=CARTESIAN_POINT('Ctrl Pts',(10.6826062055719,-1.,4.92984378812836));
#7753=CARTESIAN_POINT('Ctrl Pts',(10.7173937944281,-1.,4.92984378812836));
#7754=CARTESIAN_POINT('Ctrl Pts',(10.7360319592806,-1.0009878010724,4.9328814434269));
#7755=CARTESIAN_POINT('Ctrl Pts',(10.7711257791067,-1.0047701664708,4.9450775807219));
#7756=CARTESIAN_POINT('Ctrl Pts',(10.7875957538804,-1.00753000589576,4.954205579358));
#7757=CARTESIAN_POINT('Ctrl Pts',(10.8223106862062,-1.01472209320273,4.9796449878867));
#7758=CARTESIAN_POINT('Ctrl Pts',(10.839847070119,-1.01970376154596,4.99863134755478));
#7759=CARTESIAN_POINT('Ctrl Pts',(10.8694149146398,-1.02931935924876,5.04147273982077));
#7760=CARTESIAN_POINT('Ctrl Pts',(10.8813992178595,-1.0339550375075,5.06535990747913));
#7761=CARTESIAN_POINT('Ctrl Pts',(10.9096209325494,-1.04560657967159,5.14124876244566));
#7762=CARTESIAN_POINT('Ctrl Pts',(10.917944947177,-1.05,5.19751752176563));
#7763=CARTESIAN_POINT('Ctrl Pts',(10.917944947177,-1.05,5.30248247823437));
#7764=CARTESIAN_POINT('Ctrl Pts',(10.9096209325494,-1.04560657967159,5.35875123755434));
#7765=CARTESIAN_POINT('Ctrl Pts',(10.8813992178595,-1.0339550375075,5.43464009252087));
#7766=CARTESIAN_POINT('Ctrl Pts',(10.8694149146398,-1.02931935924876,5.45852726017923));
#7767=CARTESIAN_POINT('Ctrl Pts',(10.839847070119,-1.01970376154596,5.50136865244522));
#7768=CARTESIAN_POINT('Ctrl Pts',(10.8223106862062,-1.01472209320273,5.5203550121133));
#7769=CARTESIAN_POINT('Ctrl Pts',(10.7875957538804,-1.00753000589576,5.545794420642));
#7770=CARTESIAN_POINT('Ctrl Pts',(10.7711257791067,-1.0047701664708,5.5549224192781));
#7771=CARTESIAN_POINT('Ctrl Pts',(10.7360319592806,-1.0009878010724,5.5671185565731));
#7772=CARTESIAN_POINT('Ctrl Pts',(10.7173937944281,-1.,5.57015621187164));
#7773=CARTESIAN_POINT('Ctrl Pts',(10.6826062055719,-1.,5.57015621187164));
#7774=CARTESIAN_POINT('Ctrl Pts',(10.6639680407194,-1.0009878010724,5.5671185565731));
#7775=CARTESIAN_POINT('Ctrl Pts',(10.6288742208933,-1.0047701664708,5.5549224192781));
#7776=CARTESIAN_POINT('Ctrl Pts',(10.6124042461196,-1.00753000589576,5.545794420642));
#7777=CARTESIAN_POINT('Ctrl Pts',(10.5776893137938,-1.01472209320273,5.5203550121133));
#7778=CARTESIAN_POINT('Ctrl Pts',(10.560152929881,-1.01970376154596,5.50136865244522));
#7779=CARTESIAN_POINT('Ctrl Pts',(10.5305850853602,-1.02931935924876,5.45852726017923));
#7780=CARTESIAN_POINT('Ctrl Pts',(10.5186007821405,-1.0339550375075,5.43464009252087));
#7781=CARTESIAN_POINT('Ctrl Pts',(10.4903790674506,-1.04560657967159,5.35875123755434));
#7782=CARTESIAN_POINT('Ctrl Pts',(10.482055052823,-1.05,5.30248247823437));
#7783=CARTESIAN_POINT('Ctrl Pts',(10.482055052823,-1.05,5.25));
#7784=CARTESIAN_POINT('Origin',(10.7,-1.5,2.));
#7785=CARTESIAN_POINT('',(10.425,-1.5,2.));
#7786=CARTESIAN_POINT('Origin',(10.7,-1.5,2.));
#7787=CARTESIAN_POINT('Origin',(10.7,-1.5,0.9));
#7788=CARTESIAN_POINT('',(10.425,-1.5,1.));
#7789=CARTESIAN_POINT('Origin',(10.7,-1.5,1.));
#7790=CARTESIAN_POINT('',(10.425,-1.5,0.9));
#7791=CARTESIAN_POINT('Origin',(9.9,0.,5.25));
#7792=CARTESIAN_POINT('',(10.,-1.28587913910472E-16,6.3));
#7793=CARTESIAN_POINT('Origin',(10.,0.,5.25));
#7794=CARTESIAN_POINT('',(13.,1.28587913910472E-16,6.3));
#7795=CARTESIAN_POINT('',(9.9,-1.28587913910472E-16,6.3));
#7796=CARTESIAN_POINT('Origin',(13.,0.,5.25));
#7797=CARTESIAN_POINT('Origin',(13.,-2.,1.));
#7798=CARTESIAN_POINT('',(13.,-2.,1.));
#7799=CARTESIAN_POINT('Origin',(10.,2.,1.));
#7800=CARTESIAN_POINT('',(10.,2.,1.));
#7801=CARTESIAN_POINT('Origin',(11.5,0.,1.));
#10973=UNCERTAINTY_MEASURE_WITH_UNIT(LENGTH_MEASURE(0.001),#11036,
'DISTANCE_ACCURACY_VALUE',
'Maximum model space distance between geometric entities at asserted c
onnectivities');
#11002=UNCERTAINTY_MEASURE_WITH_UNIT(LENGTH_MEASURE(0.001),#11036,
'DISTANCE_ACCURACY_VALUE',
'Maximum model space distance between geometric entities at asserted c
onnectivities');
#11006=(
GEOMETRIC_REPRESENTATION_CONTEXT(3)
GLOBAL_UNCERTAINTY_ASSIGNED_CONTEXT((#10973))
GLOBAL_UNIT_ASSIGNED_CONTEXT((#11036,#11038,#11039))
REPRESENTATION_CONTEXT('','3D')
);
#11035=(
GEOMETRIC_REPRESENTATION_CONTEXT(3)
GLOBAL_UNCERTAINTY_ASSIGNED_CONTEXT((#11002))
GLOBAL_UNIT_ASSIGNED_CONTEXT((#11036,#11038,#11039))
REPRESENTATION_CONTEXT('','3D')
);
#11036=(
LENGTH_UNIT()
NAMED_UNIT(*)
SI_UNIT(.CENTI.,.METRE.)
);
#11038=(
NAMED_UNIT(*)
PLANE_ANGLE_UNIT()
SI_UNIT($,.RADIAN.)
);
#11039=(
NAMED_UNIT(*)
SI_UNIT($,.STERADIAN.)
SOLID_ANGLE_UNIT()
);
#11043=SHAPE_DEFINITION_REPRESENTATION(#11075,#11156);
#11075=PRODUCT_DEFINITION_SHAPE('',$,#11189);
#11156=SHAPE_REPRESENTATION('',(#5043),#11006);
#11185=PRODUCT_DEFINITION_CONTEXT('part definition',#11283,'design');
#11189=PRODUCT_DEFINITION('Linear follower guide',
'Linear follower guide',#11221,#11185);
#11221=PRODUCT_DEFINITION_FORMATION('',$,#11288);
#11283=APPLICATION_CONTEXT(
'Core Data for Automotive Mechanical Design Process');
#11284=PRODUCT_CONTEXT('part definition',#11283,'mechanical');
#11288=PRODUCT('Linear follower guide','Linear follower guide',
'Linear follower guide',(#11284));
#11394=COLOUR_RGB('Off White',0.89,0.88,0.83);
#11395=FILL_AREA_STYLE_COLOUR('',#11394);
#11396=FILL_AREA_STYLE('',(#11395));
#11397=SURFACE_STYLE_FILL_AREA(#11396);
#11398=SURFACE_SIDE_STYLE('',(#11397));
#11399=SURFACE_STYLE_USAGE(.BOTH.,#11398);
#11400=PRESENTATION_STYLE_ASSIGNMENT((#11399));
ENDSEC;
END-ISO-10303-21;
